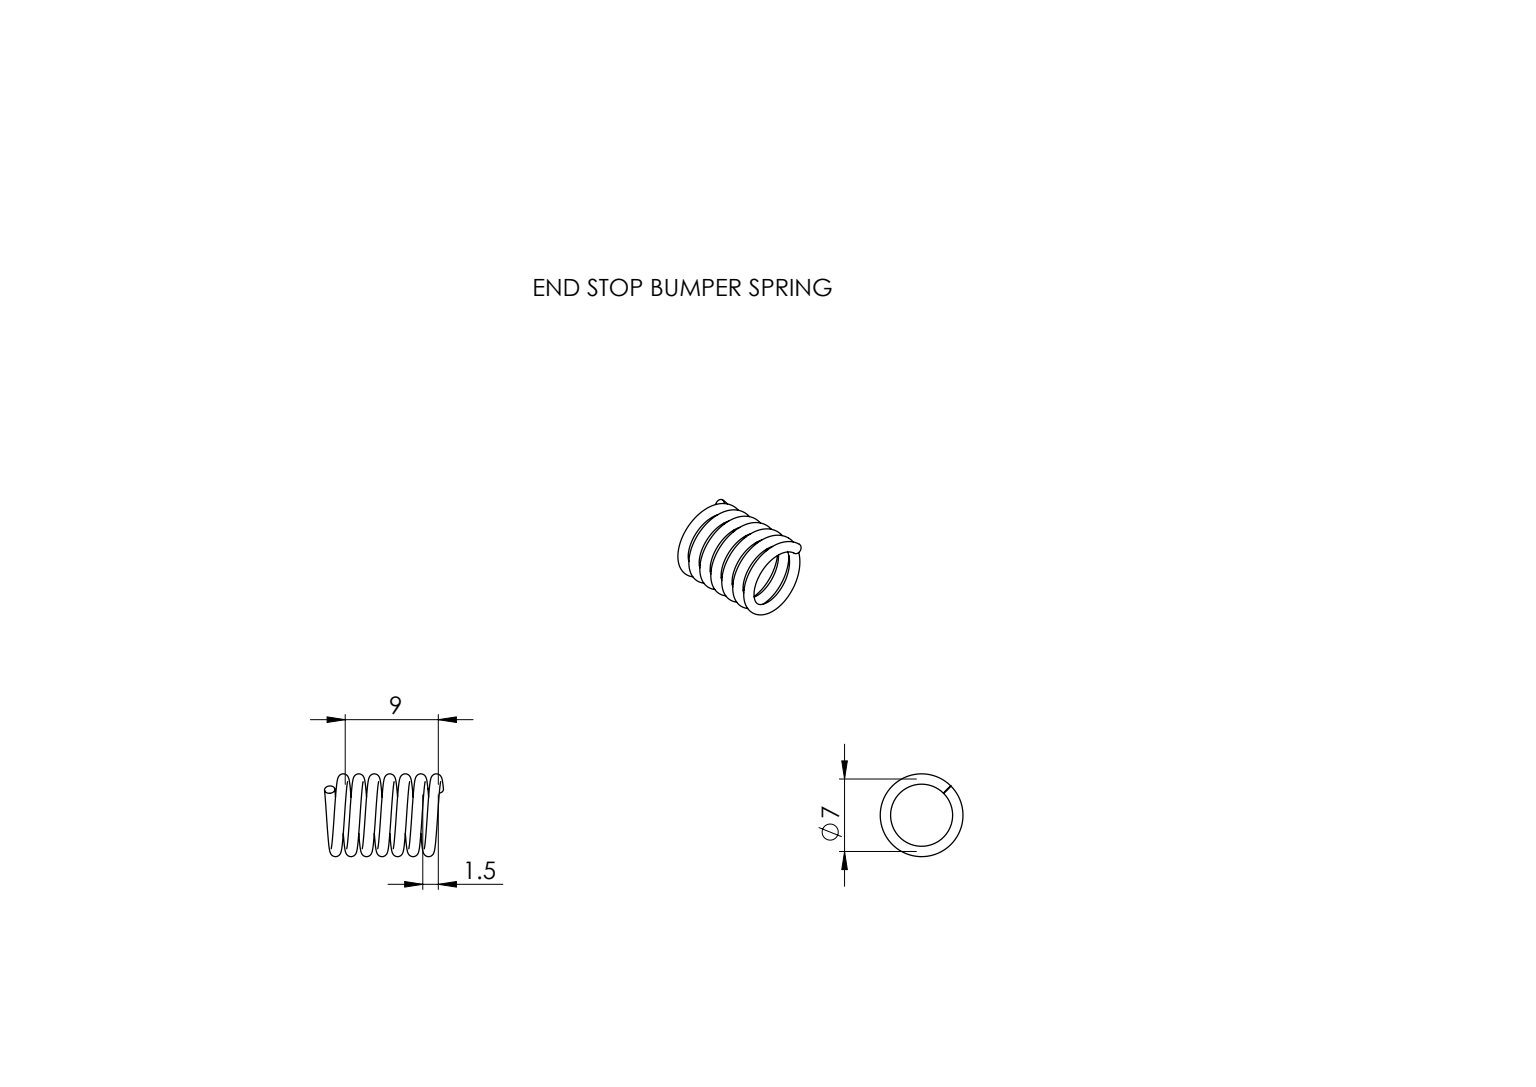
ISO-10303-21;
HEADER;
FILE_DESCRIPTION (('STEP AP214'),
    '1' );
FILE_NAME ('End Stop Bumper spring.step',
    '2026-10-08T13:46:47',
    ( '' ),
    ( '' ),
    'SwSTEP 2.0',
    'SolidWorks 2026',
    '' );
FILE_SCHEMA (( 'AUTOMOTIVE_DESIGN' ));
ENDSEC;

DATA;
#21=CARTESIAN_POINT ( 'NONE',  ( 57.71643183416158251, 13.97181229448536399, 16.72490539043799629 ) ) ;
#31=CARTESIAN_POINT ( 'NONE',  ( 51.40856816583843880, 12.97181229448534978, 13.68930817193506755 ) ) ;
#36=CARTESIAN_POINT ( 'NONE',  ( 52.87500000000000711, 7.878679656440349177, 12.87867965644035984 ) ) ;
#39=CARTESIAN_POINT ( 'NONE',  ( 51.09375000000000000, 11.24264068711927322, 11.99999999999998934 ) ) ;
#46=CARTESIAN_POINT ( 'NONE',  ( 51.56250000000000711, 6.999999999999997335, 15.00000000000000533 ) ) ;
#62=CARTESIAN_POINT ( 'NONE',  ( 52.25231816583844591, 7.219692298483957771, 17.87654654797633924 ) ) ;
#75=CARTESIAN_POINT ( 'NONE',  ( 53.43750000000000711, 10.00000000000001776, 18.99999999999999645 ) ) ;
#79=CARTESIAN_POINT ( 'NONE',  ( 56.84606816583843880, 8.411196891453267099, 19.02818770551464667 ) ) ;
#89=CARTESIAN_POINT ( 'NONE',  ( 52.27893183416158251, 8.411196891453236901, 10.97181229448535511 ) ) ;
#97=CARTESIAN_POINT ( 'NONE',  ( 53.25000000000000711, 7.878679656440361612, 17.12132034355964549 ) ) ;
#132=CARTESIAN_POINT ( 'NONE',  ( 56.49768183416158962, 12.87654654797631792, 12.21969229848393113 ) ) ;
#140=CARTESIAN_POINT ( 'NONE',  ( 50.84606816583843880, 8.825410453826357582, 18.02818770551464667 ) ) ;
#148=CARTESIAN_POINT ( 'NONE',  ( 52.59375000000000711, 11.24264068711927322, 11.99999999999998934 ) ) ;
#151=CARTESIAN_POINT ( 'NONE',  ( 53.53125000000000000, 11.24264068711929276, 18.00000000000000355 ) ) ;
#159=CARTESIAN_POINT ( 'NONE',  ( 56.53125000000000711, 11.24264068711929276, 18.00000000000000355 ) ) ;
#177=CARTESIAN_POINT ( 'NONE',  ( 52.43981816583844591, 10.06805114094564857, 19.00000000000000000 ) ) ;
#192=CARTESIAN_POINT ( 'NONE',  ( 58.59375000000000711, 11.65685424949236015, 10.99999999999998579 ) ) ;
#196=CARTESIAN_POINT ( 'NONE',  ( 54.97106816583843880, 5.971812294485345340, 13.41119689145326710 ) ) ;
#204=CARTESIAN_POINT ( 'NONE',  ( 56.49768183416158962, 12.87654654797631792, 12.21969229848393113 ) ) ;
#244=CARTESIAN_POINT ( 'NONE',  ( 55.93518183416157541, 9.931948859054379852, 18.99999999999999289 ) ) ;
#253=CARTESIAN_POINT ( 'NONE',  ( 54.56250000000000711, 6.999999999999997335, 15.00000000000000533 ) ) ;
#259=CARTESIAN_POINT ( 'NONE',  ( 59.96643183416158251, 7.028187705514638672, 13.68930817193508531 ) ) ;
#262=CARTESIAN_POINT ( 'NONE',  ( 54.28125000000000000, 8.757359312880703683, 11.99999999999999822 ) ) ;
#273=CARTESIAN_POINT ( 'NONE',  ( 56.15625000000002132, 7.000000000000003553, 16.24264068711929099 ) ) ;
#292=CARTESIAN_POINT ( 'NONE',  ( 59.00231816583843170, 12.07320092032949610, 12.83056023321021044 ) ) ;
#312=CARTESIAN_POINT ( 'NONE',  ( 54.37500000000000711, 7.171572875253794166, 12.17157287525381726 ) ) ;
#317=CARTESIAN_POINT ( 'NONE',  ( 51.78356816583844591, 8.275094609561968184, 11.02818770551464667 ) ) ;
#326=CARTESIAN_POINT ( 'NONE',  ( 53.21643183416158251, 13.97181229448536399, 16.72490539043799629 ) ) ;
#372=CARTESIAN_POINT ( 'NONE',  ( 57.18750000000000000, 9.999999999999978684, 10.99999999999999645 ) ) ;
#382=CARTESIAN_POINT ( 'NONE',  ( 53.43750000000000711, 10.00000000000000711, 17.99999999999999645 ) ) ;
#391=CARTESIAN_POINT ( 'NONE',  ( 55.65393183416158251, 6.971812294485357775, 16.17458954617365663 ) ) ;
#393=CARTESIAN_POINT ( 'NONE',  ( 55.21875000000000000, 13.00000000000000711, 16.24264068711927322 ) ) ;
#403=CARTESIAN_POINT ( 'NONE',  ( 56.31018183416157541, 12.99999999999999822, 15.06805114094562192 ) ) ;
#421=CARTESIAN_POINT ( 'NONE',  ( 54.97106816583843880, 5.971812294485345340, 13.41119689145326710 ) ) ;
#425=DIRECTION ( 'NONE',  ( 0.000000000000000000, 0.7071067811865414665, -0.7071067811865536790 ) ) ;
#440=CARTESIAN_POINT ( 'NONE',  ( 56.75231816583843170, 7.219692298483957771, 17.87654654797633924 ) ) ;
#450=CARTESIAN_POINT ( 'NONE',  ( 52.18518183416157541, 10.06805114094561659, 10.99999999999999645 ) ) ;
#454=DIRECTION ( 'NONE',  ( 0.06805114094563399774, -0.7054675904022866817, -0.7054675904022729149 ) ) ;
#493=CARTESIAN_POINT ( 'NONE',  ( 58.68750000000000000, 9.999999999999978684, 10.99999999999999645 ) ) ;
#501=CARTESIAN_POINT ( 'NONE',  ( 55.12500000000000711, 12.12132034355964727, 17.12132034355963484 ) ) ;
#508=CARTESIAN_POINT ( 'NONE',  ( 56.31018183416157541, 12.99999999999999822, 15.06805114094562192 ) ) ;
#517=CARTESIAN_POINT ( 'NONE',  ( 55.74768183416157541, 7.830560233210222876, 17.07320092032950498 ) ) ;
#534=CARTESIAN_POINT ( 'NONE',  ( 56.47106816583845301, 6.971812294485350670, 13.82541045382635403 ) ) ;
#560=CARTESIAN_POINT ( 'NONE',  ( 53.40393183416157541, 14.02818770551463956, 13.41119689145323335 ) ) ;
#568=CARTESIAN_POINT ( 'NONE',  ( 52.68750000000000711, 9.999999999999989342, 11.99999999999999467 ) ) ;
#605=CARTESIAN_POINT ( 'NONE',  ( 57.37500000000000000, 7.171572875253794166, 12.17157287525381726 ) ) ;
#608=ADVANCED_FACE ( 'NONE', ( #8331 ), #21063, .T. ) ;
#616=CARTESIAN_POINT ( 'NONE',  ( 58.50000000000000000, 12.12132034355963484, 12.87867965644034740 ) ) ;
#622=CARTESIAN_POINT ( 'NONE',  ( 54.15393183416158251, 6.971812294485357775, 16.17458954617365663 ) ) ;
#630=CARTESIAN_POINT ( 'NONE',  ( 59.87268183416157541, 7.926799079670491466, 12.83056023321021755 ) ) ;
#649=CARTESIAN_POINT ( 'NONE',  ( 53.93981816583844591, 10.06805114094563791, 17.99999999999999645 ) ) ;
#674=CARTESIAN_POINT ( 'NONE',  ( 57.09375000000000711, 11.65685424949236193, 10.99999999999998401 ) ) ;
#727=CARTESIAN_POINT ( 'NONE',  ( 58.21875000000000711, 14.00000000000000888, 16.65685424949235482 ) ) ;
#738=CARTESIAN_POINT ( 'NONE',  ( 55.50000000000000711, 12.12132034355963484, 12.87867965644034740 ) ) ;
#745=CARTESIAN_POINT ( 'NONE',  ( 57.62268183416157541, 12.07320092032950676, 17.16943976678977180 ) ) ;
#758=CARTESIAN_POINT ( 'NONE',  ( 59.77893183416158962, 8.825410453826341595, 11.97181229448535511 ) ) ;
#778=CARTESIAN_POINT ( 'NONE',  ( 54.12731816583844591, 12.16943976678978601, 17.07320092032949432 ) ) ;
#802=CARTESIAN_POINT ( 'NONE',  ( 58.68750000000000000, 9.999999999999978684, 10.99999999999999645 ) ) ;
#855=CARTESIAN_POINT ( 'NONE',  ( 55.27893183416158251, 8.825410453826341595, 11.97181229448535511 ) ) ;
#864=CARTESIAN_POINT ( 'NONE',  ( 58.46643183416158251, 7.028187705514638672, 13.68930817193508531 ) ) ;
#875=CARTESIAN_POINT ( 'NONE',  ( 57.03356816583845301, 11.31069182806492712, 17.97181229448534623 ) ) ;
#885=CARTESIAN_POINT ( 'NONE',  ( 56.00231816583843170, 12.07320092032949610, 12.83056023321021044 ) ) ;
#911=CARTESIAN_POINT ( 'NONE',  ( 54.37500000000000711, 7.171572875253794166, 12.17157287525381726 ) ) ;
#962=CARTESIAN_POINT ( 'NONE',  ( 51.75000000000000711, 7.878679656440361612, 17.12132034355964549 ) ) ;
#969=CARTESIAN_POINT ( 'NONE',  ( 60.62268183416157541, 12.78030770151606177, 17.87654654797631792 ) ) ;
#982=CARTESIAN_POINT ( 'NONE',  ( 58.65393183416157541, 5.971812294485358663, 16.58880310854675599 ) ) ;
#993=CARTESIAN_POINT ( 'NONE',  ( 50.28356816583843880, 8.275094609561968184, 11.02818770551464667 ) ) ;
#1003=CARTESIAN_POINT ( 'NONE',  ( 54.40856816583843880, 12.97181229448534978, 13.68930817193506755 ) ) ;
#1028=CARTESIAN_POINT ( 'NONE',  ( 58.78125000000000711, 8.343145750507600766, 11.00000000000000533 ) ) ;
#1086=CARTESIAN_POINT ( 'NONE',  ( 58.46643183416158251, 6.028187705514633343, 13.27509460956200016 ) ) ;
#1097=CARTESIAN_POINT ( 'NONE',  ( 60.71643183416158962, 13.97181229448536399, 16.72490539043799629 ) ) ;
#1107=CARTESIAN_POINT ( 'NONE',  ( 57.59606816583843880, 11.17458954617364242, 11.97181229448534800 ) ) ;
#1120=CARTESIAN_POINT ( 'NONE',  ( 50.93981816583844591, 10.06805114094563791, 17.99999999999999645 ) ) ;
#1148=CARTESIAN_POINT ( 'NONE',  ( 55.68750000000000000, 9.999999999999978684, 10.99999999999999645 ) ) ;
#1177=APPLICATION_CONTEXT ( 'automotive_design' ) ;
#1198=CARTESIAN_POINT ( 'NONE',  ( 51.37500000000000711, 7.878679656440349177, 12.87867965644035984 ) ) ;
#1205=CARTESIAN_POINT ( 'NONE',  ( 60.00000000000001421, 11.22198354879773419, 18.10280442057481665 ) ) ;
#1214=CARTESIAN_POINT ( 'NONE',  ( 59.68518183416157541, 10.06805114094561659, 10.99999999999999645 ) ) ;
#1223=CARTESIAN_POINT ( 'NONE',  ( 55.06481816583844591, 6.999999999999998224, 15.06805114094563436 ) ) ;
#1229=CARTESIAN_POINT ( 'NONE',  ( 59.34375000000000711, 8.757359312880723223, 18.00000000000000355 ) ) ;
#1231=CARTESIAN_POINT ( 'NONE',  ( 57.28125000000000711, 8.757359312880703683, 11.99999999999999822 ) ) ;
#1241=CARTESIAN_POINT ( 'NONE',  ( 59.25000000000000711, 7.878679656440361612, 17.12132034355964549 ) ) ;
#1257=CARTESIAN_POINT ( 'NONE',  ( 52.31250000000000711, 14.00000000000000000, 14.99999999999997691 ) ) ;
#1277=CARTESIAN_POINT ( 'NONE',  ( 51.56250000000000711, 5.999999999999996447, 15.00000000000001599 ) ) ;
#1295=CARTESIAN_POINT ( 'NONE',  ( 59.90625000000000711, 12.99999999999999645, 13.75735931288070191 ) ) ;
#1310=CARTESIAN_POINT ( 'NONE',  ( 51.18750000000000711, 9.999999999999989342, 11.99999999999999467 ) ) ;
#1328=CARTESIAN_POINT ( 'NONE',  ( 54.52893183416158962, 11.17458954617365663, 18.02818770551464311 ) ) ;
#1341=CARTESIAN_POINT ( 'NONE',  ( 50.65856816583843880, 6.028187705514649330, 16.72490539043803182 ) ) ;
#1348=CARTESIAN_POINT ( 'NONE',  ( 59.15625000000002132, 7.000000000000003553, 16.24264068711929099 ) ) ;
#1351=CARTESIAN_POINT ( 'NONE',  ( 51.50231816583844591, 12.07320092032949610, 12.83056023321021044 ) ) ;
#1360=CARTESIAN_POINT ( 'NONE',  ( 57.56250000000000000, 6.999999999999997335, 15.00000000000000533 ) ) ;
#1375=CARTESIAN_POINT ( 'NONE',  ( 56.93981816583843170, 10.06805114094564857, 19.00000000000000000 ) ) ;
#1387=CARTESIAN_POINT ( 'NONE',  ( 59.34375000000000711, 8.343145750507636293, 19.00000000000000000 ) ) ;
#1391=CARTESIAN_POINT ( 'NONE',  ( 57.68981816583843170, 9.931948859054346102, 10.99999999999999467 ) ) ;
#1410=CARTESIAN_POINT ( 'NONE',  ( 54.75000000000000711, 7.878679656440361612, 17.12132034355964549 ) ) ;
#1435=CARTESIAN_POINT ( 'NONE',  ( 60.00000000000002132, 13.28258829677531239, 17.07862169589594004 ) ) ;
#1449=CARTESIAN_POINT ( 'NONE',  ( 54.15393183416158251, 6.971812294485357775, 16.17458954617365663 ) ) ;
#1459=CARTESIAN_POINT ( 'NONE',  ( 51.12731816583844591, 12.16943976678978601, 17.07320092032949432 ) ) ;
#1469=CARTESIAN_POINT ( 'NONE',  ( 56.81250000000000000, 13.00000000000000000, 14.99999999999998757 ) ) ;
#1472=CARTESIAN_POINT ( 'NONE',  ( 50.18981816583844591, 9.931948859054354983, 11.99999999999999645 ) ) ;
#1478=VERTEX_POINT ( 'NONE', #10701 ) ;
#1482=CARTESIAN_POINT ( 'NONE',  ( 59.15625000000002132, 7.000000000000003553, 16.24264068711929099 ) ) ;
#1507=CARTESIAN_POINT ( 'NONE',  ( 51.84375000000001421, 8.343145750507638070, 19.00000000000000711 ) ) ;
#1523=CARTESIAN_POINT ( 'NONE',  ( 58.81481816583843170, 14.00000000000000178, 14.93194885905434610 ) ) ;
#1531=CARTESIAN_POINT ( 'NONE',  ( 52.93518183416157541, 9.931948859054372747, 17.99999999999999645 ) ) ;
#1540=CARTESIAN_POINT ( 'NONE',  ( 59.53125000000000711, 11.24264068711929276, 18.00000000000000000 ) ) ;
#1572=CARTESIAN_POINT ( 'NONE',  ( 56.21643183416158251, 13.97181229448536399, 16.72490539043799629 ) ) ;
#1583=CARTESIAN_POINT ( 'NONE',  ( 59.62500000000000711, 12.12132034355964727, 17.12132034355963484 ) ) ;
#1590=CARTESIAN_POINT ( 'NONE',  ( 54.65625000000001421, 7.000000000000003553, 16.24264068711929099 ) ) ;
#1592=CARTESIAN_POINT ( 'NONE',  ( 59.15625000000002132, 7.000000000000003553, 16.24264068711929099 ) ) ;
#1601=CARTESIAN_POINT ( 'NONE',  ( 55.50000000000000711, 12.12132034355963484, 12.87867965644034740 ) ) ;
#1621=CARTESIAN_POINT ( 'NONE',  ( 56.37731816583843170, 7.123453452023657206, 12.21969229848395599 ) ) ;
#1641=CARTESIAN_POINT ( 'NONE',  ( 53.62500000000000711, 12.82842712474620228, 17.82842712474617386 ) ) ;
#1650=CARTESIAN_POINT ( 'NONE',  ( 52.46643183416157541, 7.028187705514638672, 13.68930817193508531 ) ) ;
#1658=CARTESIAN_POINT ( 'NONE',  ( 56.71875000000000711, 13.00000000000000533, 16.24264068711927322 ) ) ;
#1688=CARTESIAN_POINT ( 'NONE',  ( 52.93518183416157541, 9.931948859054379852, 18.99999999999999289 ) ) ;
#1695=CARTESIAN_POINT ( 'NONE',  ( 58.87500000000000711, 7.878679656440349177, 12.87867965644035984 ) ) ;
#1703=CARTESIAN_POINT ( 'NONE',  ( 53.71875000000002132, 13.00000000000000711, 16.24264068711927322 ) ) ;
#1705=CARTESIAN_POINT ( 'NONE',  ( 52.78125000000000711, 8.757359312880703683, 11.99999999999999822 ) ) ;
#1713=CARTESIAN_POINT ( 'NONE',  ( 53.53125000000000000, 11.24264068711929276, 18.00000000000000355 ) ) ;
#1737=CARTESIAN_POINT ( 'NONE',  ( 55.34606816583843880, 8.411196891453267099, 19.02818770551464667 ) ) ;
#1740=SURFACE_STYLE_USAGE ( .BOTH. , #14468 ) ;
#1753=CARTESIAN_POINT ( 'NONE',  ( 55.87500000000000711, 7.171572875253794166, 12.17157287525381726 ) ) ;
#1757=CARTESIAN_POINT ( 'NONE',  ( 54.65625000000001421, 6.000000000000004441, 16.65685424949239390 ) ) ;
#1766=CARTESIAN_POINT ( 'NONE',  ( 57.81018183416157541, 14.00000000000000000, 15.06805114094561304 ) ) ;
#1774=CARTESIAN_POINT ( 'NONE',  ( 56.53125000000000711, 11.24264068711929276, 18.00000000000000000 ) ) ;
#1806=CARTESIAN_POINT ( 'NONE',  ( 53.21643183416158251, 13.97181229448536399, 16.72490539043799629 ) ) ;
#1814=CARTESIAN_POINT ( 'NONE',  ( 51.97106816583844591, 6.971812294485350670, 13.82541045382635403 ) ) ;
#1820=CARTESIAN_POINT ( 'NONE',  ( 55.12500000000000711, 12.12132034355964727, 17.12132034355963484 ) ) ;
#1824=CARTESIAN_POINT ( 'NONE',  ( 53.71875000000002132, 13.00000000000000711, 16.24264068711927322 ) ) ;
#1831=CARTESIAN_POINT ( 'NONE',  ( 51.93750000000000711, 10.00000000000000711, 17.99999999999999645 ) ) ;
#1851=CARTESIAN_POINT ( 'NONE',  ( 51.31481816583844591, 14.00000000000000178, 14.93194885905434610 ) ) ;
#1867=CARTESIAN_POINT ( 'NONE',  ( 53.90625000000000000, 13.99999999999999289, 13.34314575050759544 ) ) ;
#1872=CARTESIAN_POINT ( 'NONE',  ( 56.09606816583844591, 11.58880310854672935, 10.97181229448534445 ) ) ;
#1884=CARTESIAN_POINT ( 'NONE',  ( 55.27893183416158251, 8.411196891453236901, 10.97181229448535511 ) ) ;
#1893=CARTESIAN_POINT ( 'NONE',  ( 51.09375000000000711, 11.24264068711927322, 11.99999999999998934 ) ) ;
#1927=CARTESIAN_POINT ( 'NONE',  ( 58.27893183416158962, 8.411196891453236901, 10.97181229448535511 ) ) ;
#1936=CARTESIAN_POINT ( 'NONE',  ( 52.25231816583844591, 7.926799079670502124, 17.16943976678978245 ) ) ;
#1943=CARTESIAN_POINT ( 'NONE',  ( 54.28125000000000000, 8.757359312880703683, 11.99999999999999822 ) ) ;
#1946=CARTESIAN_POINT ( 'NONE',  ( 54.75000000000000711, 7.878679656440361612, 17.12132034355964549 ) ) ;
#1953=CARTESIAN_POINT ( 'NONE',  ( 52.31250000000000711, 13.00000000000000000, 14.99999999999998757 ) ) ;
#1968=CARTESIAN_POINT ( 'NONE',  ( 51.22106816583844591, 14.02818770551465377, 16.58880310854672757 ) ) ;
#1982=CARTESIAN_POINT ( 'NONE',  ( 59.06250000000000711, 5.999999999999996447, 15.00000000000001599 ) ) ;
#1986=CARTESIAN_POINT ( 'NONE',  ( 55.43981816583843170, 10.06805114094564857, 19.00000000000000000 ) ) ;
#1995=CARTESIAN_POINT ( 'NONE',  ( 59.15625000000002132, 6.000000000000004441, 16.65685424949239390 ) ) ;
#2002=CARTESIAN_POINT ( 'NONE',  ( 52.31250000000000711, 13.00000000000000000, 14.99999999999998757 ) ) ;
#2041=CARTESIAN_POINT ( 'NONE',  ( 54.15393183416158251, 5.971812294485358663, 16.58880310854675599 ) ) ;
#2047=CARTESIAN_POINT ( 'NONE',  ( 54.00000000000000711, 12.12132034355963484, 12.87867965644034740 ) ) ;
#2053=CARTESIAN_POINT ( 'NONE',  ( 55.68750000000000000, 9.999999999999989342, 11.99999999999999467 ) ) ;
#2066=CARTESIAN_POINT ( 'NONE',  ( 53.90625000000000000, 12.99999999999999645, 13.75735931288070191 ) ) ;
#2084=CARTESIAN_POINT ( 'NONE',  ( 53.75231816583844591, 7.219692298483957771, 17.87654654797633924 ) ) ;
#2088=EDGE_CURVE ( 'NONE', #16693, #10540, #5521, .T. ) ;
#2099=CARTESIAN_POINT ( 'NONE',  ( 57.28125000000000711, 8.343145750507600766, 11.00000000000000355 ) ) ;
#2103=CARTESIAN_POINT ( 'NONE',  ( 53.00231816583844591, 12.78030770151603868, 12.12345345202365188 ) ) ;
#2114=CARTESIAN_POINT ( 'NONE',  ( 54.99768183416157541, 12.87654654797631792, 12.21969229848393113 ) ) ;
#2126=EDGE_LOOP ( 'NONE', ( #8202, #17901 ) ) ;
#2156=CARTESIAN_POINT ( 'NONE',  ( 57.84375000000000711, 8.343145750507638070, 19.00000000000000711 ) ) ;
#2166=CARTESIAN_POINT ( 'NONE',  ( 55.87500000000000711, 7.878679656440349177, 12.87867965644035984 ) ) ;
#2176=CARTESIAN_POINT ( 'NONE',  ( 59.02893183416158251, 11.17458954617365663, 18.02818770551464311 ) ) ;
#2179=CARTESIAN_POINT ( 'NONE',  ( 54.93750000000000711, 10.00000000000000711, 17.99999999999999645 ) ) ;
#2189=CARTESIAN_POINT ( 'NONE',  ( 58.37268183416157541, 7.926799079670491466, 12.83056023321021755 ) ) ;
#2208=CARTESIAN_POINT ( 'NONE',  ( 53.37731816583844591, 7.123453452023657206, 12.21969229848395599 ) ) ;
#2224=CARTESIAN_POINT ( 'NONE',  ( 52.68750000000000711, 9.999999999999978684, 10.99999999999999645 ) ) ;
#2228=CARTESIAN_POINT ( 'NONE',  ( 52.90856816583843880, 13.97181229448534978, 13.27509460956196641 ) ) ;
#2240=CARTESIAN_POINT ( 'NONE',  ( 59.81250000000000711, 14.00000000000000000, 14.99999999999997691 ) ) ;
#2279=STYLED_ITEM ( 'NONE', ( #5346 ), #22323 ) ;
#2287=CARTESIAN_POINT ( 'NONE',  ( 59.15625000000002132, 6.000000000000004441, 16.65685424949239390 ) ) ;
#2297=CARTESIAN_POINT ( 'NONE',  ( 56.15625000000002132, 7.000000000000003553, 16.24264068711929099 ) ) ;
#2304=CARTESIAN_POINT ( 'NONE',  ( 58.46643183416158251, 7.028187705514638672, 13.68930817193508531 ) ) ;
#2317=CARTESIAN_POINT ( 'NONE',  ( 58.93518183416157541, 9.931948859054372747, 17.99999999999999645 ) ) ;
#2333=CARTESIAN_POINT ( 'NONE',  ( 58.06481816583843170, 6.999999999999998224, 15.06805114094563436 ) ) ;
#2360=CARTESIAN_POINT ( 'NONE',  ( 55.37268183416157541, 7.219692298483935566, 12.12345345202367675 ) ) ;
#2403=CARTESIAN_POINT ( 'NONE',  ( 55.96875000000000000, 5.999999999999987566, 13.34314575050763452 ) ) ;
#2411=CARTESIAN_POINT ( 'NONE',  ( 57.93750000000000000, 10.00000000000000711, 17.99999999999999645 ) ) ;
#2418=CARTESIAN_POINT ( 'NONE',  ( 59.77893183416158962, 8.825410453826341595, 11.97181229448535511 ) ) ;
#2427=CARTESIAN_POINT ( 'NONE',  ( 60.99768183416157541, 12.16943976678977535, 12.92679907967048614 ) ) ;
#2445=CARTESIAN_POINT ( 'NONE',  ( 57.12731816583843170, 12.16943976678978601, 17.07320092032949432 ) ) ;
#2472=CARTESIAN_POINT ( 'NONE',  ( 53.15625000000001421, 6.000000000000004441, 16.65685424949239390 ) ) ;
#2518=CARTESIAN_POINT ( 'NONE',  ( 59.90625000000000711, 13.99999999999999289, 13.34314575050759544 ) ) ;
#2522=EDGE_LOOP ( 'NONE', ( #4591, #11690 ) ) ;
#2525=CARTESIAN_POINT ( 'NONE',  ( 57.09375000000000711, 11.24264068711927322, 11.99999999999998934 ) ) ;
#2531=CARTESIAN_POINT ( 'NONE',  ( 58.56018183416157541, 7.000000000000000000, 14.93194885905437097 ) ) ;
#2540=CARTESIAN_POINT ( 'NONE',  ( 56.49768183416158962, 12.16943976678977535, 12.92679907967048614 ) ) ;
#2557=CARTESIAN_POINT ( 'NONE',  ( 56.84606816583843880, 8.825410453826357582, 18.02818770551464667 ) ) ;
#2575=CARTESIAN_POINT ( 'NONE',  ( 52.03125000000000711, 11.65685424949239923, 18.99999999999998934 ) ) ;
#2587=CARTESIAN_POINT ( 'NONE',  ( 56.25000000000000711, 7.171572875253819923, 17.82842712474619873 ) ) ;
#2657=CARTESIAN_POINT ( 'NONE',  ( 57.90393183416158251, 13.02818770551463778, 13.82541045382633982 ) ) ;
#2668=CARTESIAN_POINT ( 'NONE',  ( 59.31018183416157541, 12.99999999999999822, 15.06805114094562192 ) ) ;
#2682=CARTESIAN_POINT ( 'NONE',  ( 57.31481816583843170, 12.99999999999999822, 14.93194885905435676 ) ) ;
#2691=CARTESIAN_POINT ( 'NONE',  ( 57.68981816583843170, 9.931948859054354983, 11.99999999999999645 ) ) ;
#2713=CARTESIAN_POINT ( 'NONE',  ( 54.46875000000000000, 5.999999999999987566, 13.34314575050763452 ) ) ;
#2770=CARTESIAN_POINT ( 'NONE',  ( 53.02893183416157541, 11.17458954617365663, 18.02818770551464311 ) ) ;
#2771=CARTESIAN_POINT ( 'NONE',  ( 60.00000000000002132, 12.52638886096845816, 13.34932382114196692 ) ) ;
#2780=CARTESIAN_POINT ( 'NONE',  ( 59.40393183416158251, 14.02818770551463956, 13.41119689145323335 ) ) ;
#2791=CARTESIAN_POINT ( 'NONE',  ( 56.18981816583843170, 9.931948859054354983, 11.99999999999999645 ) ) ;
#2803=CARTESIAN_POINT ( 'NONE',  ( 54.97106816583843880, 6.971812294485350670, 13.82541045382635403 ) ) ;
#2827=CARTESIAN_POINT ( 'NONE',  ( 53.53125000000000000, 11.65685424949239923, 18.99999999999998934 ) ) ;
#2881=CARTESIAN_POINT ( 'NONE',  ( 58.37268183416157541, 7.219692298483935566, 12.12345345202367675 ) ) ;
#2893=CARTESIAN_POINT ( 'NONE',  ( 54.71643183416158251, 12.97181229448535689, 16.31069182806490758 ) ) ;
#2904=CARTESIAN_POINT ( 'NONE',  ( 58.15856816583844591, 7.028187705514647554, 16.31069182806492179 ) ) ;
#2910=CARTESIAN_POINT ( 'NONE',  ( 56.34375000000000711, 8.757359312880723223, 18.00000000000000355 ) ) ;
#2913=CARTESIAN_POINT ( 'NONE',  ( 51.68981816583844591, 9.931948859054354983, 11.99999999999999645 ) ) ;
#2940=CARTESIAN_POINT ( 'NONE',  ( 53.81250000000000711, 14.00000000000000000, 14.99999999999997691 ) ) ;
#3003=CARTESIAN_POINT ( 'NONE',  ( 60.00000000000005684, 13.02863400130356375, 14.80978507604997851 ) ) ;
#3013=CARTESIAN_POINT ( 'NONE',  ( 54.81018183416157541, 12.99999999999999822, 15.06805114094562192 ) ) ;
#3023=ORIENTED_EDGE ( 'NONE', *, *, #17689, .T. ) ;
#3024=CARTESIAN_POINT ( 'NONE',  ( 59.00231816583843170, 12.07320092032949610, 12.83056023321021044 ) ) ;
#3026=MECHANICAL_DESIGN_GEOMETRIC_PRESENTATION_REPRESENTATION('',(#8030),#3797);
#3040=CARTESIAN_POINT ( 'NONE',  ( 59.34375000000000711, 8.757359312880723223, 18.00000000000000355 ) ) ;
#3072=CARTESIAN_POINT ( 'NONE',  ( 56.47106816583845301, 5.971812294485345340, 13.41119689145326710 ) ) ;
#3087=CARTESIAN_POINT ( 'NONE',  ( 59.81250000000000711, 14.00000000000000000, 14.99999999999997691 ) ) ;
#3091=CARTESIAN_POINT ( 'NONE',  ( 54.93750000000000711, 10.00000000000001776, 18.99999999999999645 ) ) ;
#3109=CARTESIAN_POINT ( 'NONE',  ( 59.15625000000001421, 7.000000000000002665, 16.24264068711929099 ) ) ;
#3111=CARTESIAN_POINT ( 'NONE',  ( 0.000000000000000000, 0.000000000000000000, 0.000000000000000000 ) ) ;
#3137=CARTESIAN_POINT ( 'NONE',  ( 60.90393183416158962, 14.02818770551463956, 13.41119689145323335 ) ) ;
#3146=CARTESIAN_POINT ( 'NONE',  ( 54.78356816583844591, 8.689308171935074654, 12.02818770551464489 ) ) ;
#3152=CARTESIAN_POINT ( 'NONE',  ( 58.03125000000000711, 11.24264068711929276, 18.00000000000000355 ) ) ;
#3154=CARTESIAN_POINT ( 'NONE',  ( 60.00000000000000711, 12.12132034355963484, 12.87867965644034740 ) ) ;
#3162=CARTESIAN_POINT ( 'NONE',  ( 57.65625000000002132, 7.000000000000003553, 16.24264068711929099 ) ) ;
#3163=SURFACE_SIDE_STYLE ('',( #8345 ) ) ;
#3183=CARTESIAN_POINT ( 'NONE',  ( 56.84606816583843880, 8.411196891453267099, 19.02818770551464667 ) ) ;
#3198=CARTESIAN_POINT ( 'NONE',  ( 59.53125000000000711, 11.65685424949239923, 18.99999999999998934 ) ) ;
#3202=CARTESIAN_POINT ( 'NONE',  ( 55.40625000000000000, 13.99999999999999289, 13.34314575050759544 ) ) ;
#3219=CARTESIAN_POINT ( 'NONE',  ( 56.06250000000000000, 6.999999999999997335, 15.00000000000000533 ) ) ;
#3231=ORIENTED_EDGE ( 'NONE', *, *, #2088, .F. ) ;
#3246=CARTESIAN_POINT ( 'NONE',  ( 59.99999999999182165, 10.93426768979392349, 18.41713329524482390 ) ) ;
#3255=CARTESIAN_POINT ( 'NONE',  ( 59.59143183416158962, 11.72490539043799984, 11.02818770551463246 ) ) ;
#3267=CARTESIAN_POINT ( 'NONE',  ( 53.37731816583844591, 7.830560233210212218, 12.92679907967049679 ) ) ;
#3276=CARTESIAN_POINT ( 'NONE',  ( 55.96875000000000000, 6.999999999999992895, 13.75735931288071967 ) ) ;
#3278=CARTESIAN_POINT ( 'NONE',  ( 57.93750000000000000, 10.00000000000000711, 17.99999999999999645 ) ) ;
#3287=CARTESIAN_POINT ( 'NONE',  ( 58.68750000000000000, 9.999999999999989342, 11.99999999999999467 ) ) ;
#3294=FACE_OUTER_BOUND ( 'NONE', #10599, .T. ) ;
#3304=CARTESIAN_POINT ( 'NONE',  ( 51.37500000000000711, 7.171572875253794166, 12.17157287525381726 ) ) ;
#3321=CARTESIAN_POINT ( 'NONE',  ( 51.93750000000000711, 10.00000000000001776, 18.99999999999999645 ) ) ;
#3332=CARTESIAN_POINT ( 'NONE',  ( 60.24768183416157541, 7.123453452023678523, 17.78030770151605822 ) ) ;
#3342=CARTESIAN_POINT ( 'NONE',  ( 57.00000000000000000, 12.12132034355963484, 12.87867965644034740 ) ) ;
#3364=CARTESIAN_POINT ( 'NONE',  ( 60.00000000000000711, 12.67839003132778686, 16.61512380723988258 ) ) ;
#3378=CARTESIAN_POINT ( 'NONE',  ( 56.96643183416158251, 6.028187705514633343, 13.27509460956200016 ) ) ;
#3386=CARTESIAN_POINT ( 'NONE',  ( 59.90625000000000711, 12.99999999999999645, 13.75735931288070191 ) ) ;
#3393=CARTESIAN_POINT ( 'NONE',  ( 55.78125000000000000, 8.757359312880703683, 11.99999999999999822 ) ) ;
#3395=CARTESIAN_POINT ( 'NONE',  ( 50.37731816583844591, 7.830560233210212218, 12.92679907967049679 ) ) ;
#3429=CARTESIAN_POINT ( 'NONE',  ( 59.00231816583843170, 12.78030770151603868, 12.12345345202365188 ) ) ;
#3449=CARTESIAN_POINT ( 'NONE',  ( 53.53125000000000000, 11.65685424949239923, 18.99999999999998934 ) ) ;
#3458=CARTESIAN_POINT ( 'NONE',  ( 57.15393183416157541, 5.971812294485358663, 16.58880310854675599 ) ) ;
#3466=CARTESIAN_POINT ( 'NONE',  ( 54.65625000000000711, 7.000000000000002665, 16.24264068711929099 ) ) ;
#3488=CARTESIAN_POINT ( 'NONE',  ( 60.00000000000001421, 11.91318284588047405, 17.59430459896656629 ) ) ;
#3499=CARTESIAN_POINT ( 'NONE',  ( 53.31018183416157541, 14.00000000000000000, 15.06805114094561304 ) ) ;
#3508=CARTESIAN_POINT ( 'NONE',  ( 54.12731816583844591, 12.16943976678978601, 17.07320092032949432 ) ) ;
#3515=CARTESIAN_POINT ( 'NONE',  ( 55.50000000000000711, 12.12132034355963484, 12.87867965644034740 ) ) ;
#3517=CARTESIAN_POINT ( 'NONE',  ( 56.15625000000002132, 7.000000000000003553, 16.24264068711929099 ) ) ;
#3525=CARTESIAN_POINT ( 'NONE',  ( 52.59375000000000711, 11.24264068711927322, 11.99999999999998934 ) ) ;
#3542=CARTESIAN_POINT ( 'NONE',  ( 55.81481816583843170, 14.00000000000000178, 14.93194885905434610 ) ) ;
#3554=CARTESIAN_POINT ( 'NONE',  ( 58.87500000000000711, 7.171572875253794166, 12.17157287525381726 ) ) ;
#3559=CARTESIAN_POINT ( 'NONE',  ( 51.37500000000000711, 7.171572875253794166, 12.17157287525381726 ) ) ;
#3569=CARTESIAN_POINT ( 'NONE',  ( 59.40393183416158251, 14.02818770551463956, 13.41119689145323335 ) ) ;
#3577=CARTESIAN_POINT ( 'NONE',  ( 58.68750000000000000, 9.999999999999989342, 11.99999999999999467 ) ) ;
#3605=CARTESIAN_POINT ( 'NONE',  ( 52.46643183416157541, 6.028187705514633343, 13.27509460956200016 ) ) ;
#3613=CARTESIAN_POINT ( 'NONE',  ( 53.09606816583843170, 11.17458954617364242, 11.97181229448534800 ) ) ;
#3620=CARTESIAN_POINT ( 'NONE',  ( 53.15625000000001421, 7.000000000000003553, 16.24264068711929099 ) ) ;
#3623=CARTESIAN_POINT ( 'NONE',  ( 52.12500000000000711, 12.12132034355964727, 17.12132034355963484 ) ) ;
#3631=CARTESIAN_POINT ( 'NONE',  ( 54.46875000000000000, 6.999999999999992895, 13.75735931288071967 ) ) ;
#3651=CARTESIAN_POINT ( 'NONE',  ( 51.78356816583844591, 8.275094609561968184, 11.02818770551464667 ) ) ;
#3667=CARTESIAN_POINT ( 'NONE',  ( 54.00000000000000711, 12.82842712474617741, 12.17157287525379239 ) ) ;
#3671=CARTESIAN_POINT ( 'NONE',  ( 51.97106816583844591, 5.971812294485345340, 13.41119689145326710 ) ) ;
#3679=CARTESIAN_POINT ( 'NONE',  ( 52.37268183416157541, 7.219692298483935566, 12.12345345202367675 ) ) ;
#3686=CARTESIAN_POINT ( 'NONE',  ( 51.46875000000000711, 6.999999999999992006, 13.75735931288071967 ) ) ;
#3719=CARTESIAN_POINT ( 'NONE',  ( 57.43518183416157541, 9.931948859054379852, 18.99999999999999289 ) ) ;
#3729=CARTESIAN_POINT ( 'NONE',  ( 54.22106816583844591, 13.02818770551464489, 16.17458954617363531 ) ) ;
#3736=CARTESIAN_POINT ( 'NONE',  ( 51.18750000000000711, 9.999999999999989342, 11.99999999999999467 ) ) ;
#3740=CARTESIAN_POINT ( 'NONE',  ( 53.62500000000000711, 12.12132034355964727, 17.12132034355963484 ) ) ;
#3747=CARTESIAN_POINT ( 'NONE',  ( 53.34375000000000000, 8.757359312880723223, 18.00000000000000355 ) ) ;
#3770=CARTESIAN_POINT ( 'NONE',  ( 52.06481816583844591, 5.999999999999996447, 15.06805114094564502 ) ) ;
#3787=CARTESIAN_POINT ( 'NONE',  ( 58.12500000000000000, 12.82842712474620228, 17.82842712474617386 ) ) ;
#3792=CARTESIAN_POINT ( 'NONE',  ( 55.15856816583844591, 6.028187705514649330, 16.72490539043803182 ) ) ;
#3797=( GEOMETRIC_REPRESENTATION_CONTEXT ( 3 ) GLOBAL_UNCERTAINTY_ASSIGNED_CONTEXT ( ( #17687 ) ) GLOBAL_UNIT_ASSIGNED_CONTEXT ( ( #19455, #6773, #14089 ) ) REPRESENTATION_CONTEXT ( 'NONE', 'WORKASPACE' ) );
#3804=APPLICATION_CONTEXT ( 'automotive_design' ) ;
#3806=CARTESIAN_POINT ( 'NONE',  ( 60.00000000000000711, 12.82842712474617741, 12.17157287525379239 ) ) ;
#3815=CARTESIAN_POINT ( 'NONE',  ( 51.37500000000000711, 7.878679656440349177, 12.87867965644035984 ) ) ;
#3851=CARTESIAN_POINT ( 'NONE',  ( 55.27893183416158251, 8.411196891453236901, 10.97181229448535511 ) ) ;
#3859=CARTESIAN_POINT ( 'NONE',  ( 57.56250000000000000, 6.999999999999997335, 15.00000000000000533 ) ) ;
#3865=CARTESIAN_POINT ( 'NONE',  ( 54.93750000000000711, 10.00000000000000711, 17.99999999999999645 ) ) ;
#3868=CARTESIAN_POINT ( 'NONE',  ( 51.28125000000000000, 8.757359312880703683, 11.99999999999999822 ) ) ;
#3875=CARTESIAN_POINT ( 'NONE',  ( 52.96875000000000000, 6.999999999999992895, 13.75735931288071967 ) ) ;
#3889=CARTESIAN_POINT ( 'NONE',  ( 50.28356816583843880, 8.275094609561968184, 11.02818770551464667 ) ) ;
#3904=CARTESIAN_POINT ( 'NONE',  ( 55.50000000000000711, 12.82842712474617741, 12.17157287525379239 ) ) ;
#3907=CARTESIAN_POINT ( 'NONE',  ( 52.34606816583843880, 8.411196891453267099, 19.02818770551464667 ) ) ;
#3915=CARTESIAN_POINT ( 'NONE',  ( 56.77893183416158251, 8.411196891453236901, 10.97181229448535511 ) ) ;
#3965=CARTESIAN_POINT ( 'NONE',  ( 59.25000000000000711, 7.171572875253819923, 17.82842712474619873 ) ) ;
#3967=SHAPE_DEFINITION_REPRESENTATION ( #22514, #10226 ) ;
#3975=CARTESIAN_POINT ( 'NONE',  ( 58.40625000000000711, 12.99999999999999645, 13.75735931288070191 ) ) ;
#3981=CARTESIAN_POINT ( 'NONE',  ( 54.46875000000000000, 6.999999999999992895, 13.75735931288071967 ) ) ;
#3992=CARTESIAN_POINT ( 'NONE',  ( 58.09143183416158962, 11.31069182806491291, 12.02818770551463778 ) ) ;
#4011=CARTESIAN_POINT ( 'NONE',  ( 58.43981816583843170, 10.06805114094563791, 17.99999999999999645 ) ) ;
#4027=CARTESIAN_POINT ( 'NONE',  ( 58.31250000000000000, 14.00000000000000000, 14.99999999999997691 ) ) ;
#4031=CARTESIAN_POINT ( 'NONE',  ( 54.03356816583844591, 11.72490539043803004, 18.97181229448534268 ) ) ;
#4043=CARTESIAN_POINT ( 'NONE',  ( 52.56018183416157541, 5.999999999999996447, 14.93194885905437808 ) ) ;
#4051=CARTESIAN_POINT ( 'NONE',  ( 51.75000000000000711, 7.878679656440361612, 17.12132034355964549 ) ) ;
#4084=CARTESIAN_POINT ( 'NONE',  ( 58.87500000000000711, 7.171572875253794166, 12.17157287525381726 ) ) ;
#4092=CARTESIAN_POINT ( 'NONE',  ( 52.96875000000000000, 6.999999999999992895, 13.75735931288071967 ) ) ;
#4101=CARTESIAN_POINT ( 'NONE',  ( 55.37268183416157541, 7.926799079670491466, 12.83056023321021755 ) ) ;
#4113=CARTESIAN_POINT ( 'NONE',  ( 55.93518183416157541, 9.931948859054372747, 17.99999999999999645 ) ) ;
#4132=CARTESIAN_POINT ( 'NONE',  ( 55.06481816583844591, 5.999999999999996447, 15.06805114094564502 ) ) ;
#4151=CARTESIAN_POINT ( 'NONE',  ( 52.15856816583843880, 6.028187705514649330, 16.72490539043803182 ) ) ;
#4160=CIRCLE ( 'NONE', #16028, 0.5000000000000006661 ) ;
#4161=CARTESIAN_POINT ( 'NONE',  ( 56.12268183416157541, 12.78030770151606177, 17.87654654797631792 ) ) ;
#4208=CARTESIAN_POINT ( 'NONE',  ( 57.93750000000000000, 10.00000000000001776, 18.99999999999999645 ) ) ;
#4219=CARTESIAN_POINT ( 'NONE',  ( 53.25000000000000711, 7.878679656440361612, 17.12132034355964549 ) ) ;
#4226=CARTESIAN_POINT ( 'NONE',  ( 54.71643183416158251, 12.97181229448535689, 16.31069182806490758 ) ) ;
#4237=CARTESIAN_POINT ( 'NONE',  ( 57.43518183416157541, 9.931948859054372747, 17.99999999999999645 ) ) ;
#4241=ADVANCED_FACE ( 'NONE', ( #4639 ), #20680, .F. ) ;
#4257=CARTESIAN_POINT ( 'NONE',  ( 57.31481816583843170, 12.99999999999999822, 14.93194885905435676 ) ) ;
#4271=CARTESIAN_POINT ( 'NONE',  ( 52.12500000000000711, 12.82842712474620228, 17.82842712474617386 ) ) ;
#4282=CARTESIAN_POINT ( 'NONE',  ( 55.96875000000000000, 5.999999999999987566, 13.34314575050763452 ) ) ;
#4323=CARTESIAN_POINT ( 'NONE',  ( 55.50000000000000711, 12.82842712474617741, 12.17157287525379239 ) ) ;
#4331=CARTESIAN_POINT ( 'NONE',  ( 55.78125000000000000, 8.757359312880703683, 11.99999999999999822 ) ) ;
#4338=CARTESIAN_POINT ( 'NONE',  ( 59.68518183416157541, 10.06805114094562548, 11.99999999999999645 ) ) ;
#4339=CARTESIAN_POINT ( 'NONE',  ( 60.00000000000000000, 12.92210812677098275, 14.19519413938285268 ) ) ;
#4349=CARTESIAN_POINT ( 'NONE',  ( 60.43518183416157541, 9.931948859054372747, 17.99999999999999645 ) ) ;
#4368=CARTESIAN_POINT ( 'NONE',  ( 56.56481816583843170, 6.999999999999998224, 15.06805114094563436 ) ) ;
#4396=CARTESIAN_POINT ( 'NONE',  ( 57.56250000000000000, 5.999999999999996447, 15.00000000000001599 ) ) ;
#4450=CARTESIAN_POINT ( 'NONE',  ( 51.65625000000000711, 7.000000000000003553, 16.24264068711929099 ) ) ;
#4455=CARTESIAN_POINT ( 'NONE',  ( 57.52893183416158962, 11.17458954617365663, 18.02818770551464311 ) ) ;
#4464=CARTESIAN_POINT ( 'NONE',  ( 58.74768183416157541, 7.830560233210222876, 17.07320092032950498 ) ) ;
#4484=CARTESIAN_POINT ( 'NONE',  ( 55.53356816583845301, 11.31069182806492712, 17.97181229448534623 ) ) ;
#4514=CARTESIAN_POINT ( 'NONE',  ( 55.03125000000000000, 11.65685424949239923, 18.99999999999998934 ) ) ;
#4574=CARTESIAN_POINT ( 'NONE',  ( 51.09375000000000000, 11.24264068711927322, 11.99999999999998934 ) ) ;
#4581=CARTESIAN_POINT ( 'NONE',  ( 56.96643183416158251, 7.028187705514638672, 13.68930817193508531 ) ) ;
#4591=ORIENTED_EDGE ( 'NONE', *, *, #8075, .F. ) ;
#4592=CARTESIAN_POINT ( 'NONE',  ( 52.65393183416158251, 6.971812294485357775, 16.17458954617365663 ) ) ;
#4604=CARTESIAN_POINT ( 'NONE',  ( 58.72106816583844591, 13.02818770551464489, 16.17458954617363531 ) ) ;
#4615=CARTESIAN_POINT ( 'NONE',  ( 52.43981816583844591, 10.06805114094563791, 17.99999999999999645 ) ) ;
#4628=CARTESIAN_POINT ( 'NONE',  ( 51.75000000000000711, 7.171572875253819923, 17.82842712474619873 ) ) ;
#4637=CARTESIAN_POINT ( 'NONE',  ( 58.87500000000000711, 7.171572875253794166, 12.17157287525381726 ) ) ;
#4639=FACE_OUTER_BOUND ( 'NONE', #2126, .T. ) ;
#4694=CARTESIAN_POINT ( 'NONE',  ( 60.15393183416158962, 5.971812294485358663, 16.58880310854675599 ) ) ;
#4706=CARTESIAN_POINT ( 'NONE',  ( 52.37268183416157541, 7.926799079670491466, 12.83056023321021755 ) ) ;
#4716=CARTESIAN_POINT ( 'NONE',  ( 57.87731816583843170, 7.830560233210212218, 12.92679907967049679 ) ) ;
#4722=CARTESIAN_POINT ( 'NONE',  ( 58.59375000000000711, 11.24264068711927322, 11.99999999999998934 ) ) ;
#4726=CARTESIAN_POINT ( 'NONE',  ( 57.87731816583843170, 7.830560233210212218, 12.92679907967049679 ) ) ;
#4750=CARTESIAN_POINT ( 'NONE',  ( 53.34375000000000000, 8.343145750507638070, 19.00000000000000711 ) ) ;
#4807=CARTESIAN_POINT ( 'NONE',  ( 59.99999999999995026, 12.78483204250637328, 17.66020603153145885 ) ) ;
#4818=CARTESIAN_POINT ( 'NONE',  ( 53.40393183416157541, 13.02818770551463778, 13.82541045382633982 ) ) ;
#4828=CARTESIAN_POINT ( 'NONE',  ( 57.22106816583844591, 13.02818770551464489, 16.17458954617363531 ) ) ;
#4836=CARTESIAN_POINT ( 'NONE',  ( 59.81250000000000711, 13.00000000000000000, 14.99999999999998757 ) ) ;
#4839=CARTESIAN_POINT ( 'NONE',  ( 51.40856816583843880, 12.97181229448534978, 13.68930817193506755 ) ) ;
#4868=CARTESIAN_POINT ( 'NONE',  ( 58.43981816583843170, 10.06805114094564857, 19.00000000000000000 ) ) ;
#4887=CARTESIAN_POINT ( 'NONE',  ( 51.09375000000000000, 11.65685424949236193, 10.99999999999998401 ) ) ;
#4929=CARTESIAN_POINT ( 'NONE',  ( 60.00000000000000000, 13.23725887712638283, 12.63247214140022123 ) ) ;
#4940=CARTESIAN_POINT ( 'NONE',  ( 60.24768183416157541, 7.123453452023678523, 17.78030770151605822 ) ) ;
#4952=CARTESIAN_POINT ( 'NONE',  ( 51.50231816583844591, 12.78030770151603868, 12.12345345202365188 ) ) ;
#4966=CARTESIAN_POINT ( 'NONE',  ( 50.75231816583844591, 7.926799079670502124, 17.16943976678978245 ) ) ;
#4995=CARTESIAN_POINT ( 'NONE',  ( 58.72106816583844591, 14.02818770551465377, 16.58880310854672757 ) ) ;
#4996=EDGE_CURVE ( 'NONE', #16693, #8676, #18626, .T. ) ;
#5010=CARTESIAN_POINT ( 'NONE',  ( 59.62500000000000711, 12.82842712474620228, 17.82842712474617386 ) ) ;
#5014=CARTESIAN_POINT ( 'NONE',  ( 57.97106816583845301, 5.971812294485345340, 13.41119689145326710 ) ) ;
#5029=CARTESIAN_POINT ( 'NONE',  ( 56.81250000000000000, 13.00000000000000000, 14.99999999999998757 ) ) ;
#5047=CARTESIAN_POINT ( 'NONE',  ( 60.00000000000002132, 13.01044786497014805, 14.65336842865874267 ) ) ;
#5056=CARTESIAN_POINT ( 'NONE',  ( 53.49768183416157541, 12.16943976678977535, 12.92679907967048614 ) ) ;
#5066=CARTESIAN_POINT ( 'NONE',  ( 57.50231816583843170, 12.07320092032949610, 12.83056023321021044 ) ) ;
#5074=CARTESIAN_POINT ( 'NONE',  ( 56.25000000000000711, 7.878679656440361612, 17.12132034355964549 ) ) ;
#5076=CARTESIAN_POINT ( 'NONE',  ( 51.59606816583843170, 11.17458954617364242, 11.97181229448534800 ) ) ;
#5083=CARTESIAN_POINT ( 'NONE',  ( 58.59375000000000711, 11.24264068711927322, 11.99999999999998934 ) ) ;
#5104=CARTESIAN_POINT ( 'NONE',  ( 51.56250000000000711, 5.999999999999996447, 15.00000000000001599 ) ) ;
#5122=CARTESIAN_POINT ( 'NONE',  ( 51.18750000000000711, 9.999999999999978684, 10.99999999999999645 ) ) ;
#5131=CARTESIAN_POINT ( 'NONE',  ( 52.56018183416157541, 7.000000000000000000, 14.93194885905437097 ) ) ;
#5140=CARTESIAN_POINT ( 'NONE',  ( 57.46875000000000711, 6.999999999999992006, 13.75735931288071967 ) ) ;
#5173=CARTESIAN_POINT ( 'NONE',  ( 55.56018183416157541, 5.999999999999996447, 14.93194885905437808 ) ) ;
#5182=CARTESIAN_POINT ( 'NONE',  ( 50.37731816583844591, 7.830560233210212218, 12.92679907967049679 ) ) ;
#5190=CARTESIAN_POINT ( 'NONE',  ( 57.09375000000000711, 11.24264068711927322, 11.99999999999998934 ) ) ;
#5192=CARTESIAN_POINT ( 'NONE',  ( 56.34375000000000711, 8.757359312880723223, 18.00000000000000355 ) ) ;
#5202=CARTESIAN_POINT ( 'NONE',  ( 57.37500000000000000, 7.878679656440349177, 12.87867965644035984 ) ) ;
#5218=CARTESIAN_POINT ( 'NONE',  ( 51.09375000000000000, 11.65685424949236193, 10.99999999999998401 ) ) ;
#5220=FILL_AREA_STYLE ('',( #21613 ) ) ;
#5238=CARTESIAN_POINT ( 'NONE',  ( 52.96875000000000000, 5.999999999999987566, 13.34314575050763452 ) ) ;
#5248=CARTESIAN_POINT ( 'NONE',  ( 58.84143183416158962, 8.275094609562001935, 18.97181229448536044 ) ) ;
#5259=CARTESIAN_POINT ( 'NONE',  ( 55.50000000000000711, 12.12132034355963484, 12.87867965644034740 ) ) ;
#5295=CARTESIAN_POINT ( 'NONE',  ( 54.71643183416158251, 13.97181229448536399, 16.72490539043799629 ) ) ;
#5305=CARTESIAN_POINT ( 'NONE',  ( 52.34606816583843880, 8.825410453826357582, 18.02818770551464667 ) ) ;
#5312=CARTESIAN_POINT ( 'NONE',  ( 53.53125000000000000, 11.24264068711929276, 18.00000000000000355 ) ) ;
#5314=CARTESIAN_POINT ( 'NONE',  ( 58.31250000000000000, 13.00000000000000000, 14.99999999999998757 ) ) ;
#5324=CARTESIAN_POINT ( 'NONE',  ( 55.78125000000000000, 8.757359312880703683, 11.99999999999999822 ) ) ;
#5344=CARTESIAN_POINT ( 'NONE',  ( 58.06481816583843170, 5.999999999999996447, 15.06805114094564502 ) ) ;
#5346=PRESENTATION_STYLE_ASSIGNMENT (( #1740 ) ) ;
#5359=CARTESIAN_POINT ( 'NONE',  ( 56.71875000000000711, 14.00000000000001066, 16.65685424949235482 ) ) ;
#5363=CARTESIAN_POINT ( 'NONE',  ( 52.12500000000000711, 12.82842712474620228, 17.82842712474617386 ) ) ;
#5373=CARTESIAN_POINT ( 'NONE',  ( 53.49768183416157541, 12.16943976678977535, 12.92679907967048614 ) ) ;
#5383=CARTESIAN_POINT ( 'NONE',  ( 59.25000000000000711, 7.878679656440361612, 17.12132034355964549 ) ) ;
#5414=CARTESIAN_POINT ( 'NONE',  ( 52.56018183416157541, 5.999999999999996447, 14.93194885905437808 ) ) ;
#5422=CARTESIAN_POINT ( 'NONE',  ( 54.03356816583844591, 11.31069182806492712, 17.97181229448534623 ) ) ;
#5430=CARTESIAN_POINT ( 'NONE',  ( 51.37500000000000711, 7.878679656440349177, 12.87867965644035984 ) ) ;
#5433=CARTESIAN_POINT ( 'NONE',  ( 55.50000000000000711, 12.12132034355963484, 12.87867965644034740 ) ) ;
#5440=CARTESIAN_POINT ( 'NONE',  ( 52.21875000000002842, 13.00000000000000711, 16.24264068711927322 ) ) ;
#5459=CARTESIAN_POINT ( 'NONE',  ( 51.97106816583844591, 5.971812294485345340, 13.41119689145326710 ) ) ;
#5471=CARTESIAN_POINT ( 'NONE',  ( 54.56250000000000711, 5.999999999999996447, 15.00000000000001599 ) ) ;
#5476=CARTESIAN_POINT ( 'NONE',  ( 52.62731816583844591, 12.87654654797634102, 17.78030770151602979 ) ) ;
#5486=CARTESIAN_POINT ( 'NONE',  ( 54.34143183416158251, 8.275094609562001935, 18.97181229448536044 ) ) ;
#5496=CARTESIAN_POINT ( 'NONE',  ( 53.34375000000000000, 8.757359312880723223, 18.00000000000000711 ) ) ;
#5513=CARTESIAN_POINT ( 'NONE',  ( 60.00000000000000711, 12.82842712474617741, 12.17157287525379239 ) ) ;
#5521=B_SPLINE_CURVE_WITH_KNOTS ( 'NONE', 3,
 ( #7950, #6150, #2771, #10112, #4339, #5047, #3003, #21193, #8898, #6619, #12380, #23480, #16194, #3364, #7094, #12625, #3488, #14172, #15955, #1205, #19645, #10354, #21551, #15849, #19887, #19405, #23237, #8657, #3246, #17751, #13937, #21433, #6847, #23014, #8542, #14290, #14411, #4807, #21307, #1435, #14042, #12139, #10592, #17863, #12505, #17644, #21672, #8776, #23121, #12266, #6734, #16081, #23368, #4929, #19762, #19531 ),
 .UNSPECIFIED., .F., .F.,
 ( 4, 2, 2, 2, 2, 2, 2, 2, 2, 2, 2, 2, 2, 2, 2, 2, 2, 2, 2, 2, 2, 2, 2, 2, 2, 2, 2, 4 ),
 ( 0.000000000000000000, 0.0009277918325622039331, 0.001855583665124407866, 0.002319479581405509399, 0.002783375497686610932, 0.003247271413967717235, 0.003711167330248823972, 0.004638959162811037013, 0.005566750995373249619, 0.006030646911654353320, 0.006262594869794909508, 0.006378568848865185867, 0.006494542827935463093, 0.006552529817470603875, 0.006610516807005745524, 0.006726490786076029689, 0.006958438744216604091, 0.007422334660497751160, 0.008350126493060048768, 0.009277918325622346377, 0.009741814241903491711, 0.01020571015818463531, 0.01113350199074691731, 0.01206129382330919410, 0.01298908565587147089, 0.01345298157215261102, 0.01391687748843375289, 0.01484466932099604008 ),
 .UNSPECIFIED. ) ;
#5526=CARTESIAN_POINT ( 'NONE',  ( 58.09143183416158962, 11.72490539043799984, 11.02818770551463246 ) ) ;
#5535=CARTESIAN_POINT ( 'NONE',  ( 52.53356816583844591, 11.31069182806492712, 17.97181229448534623 ) ) ;
#5543=CARTESIAN_POINT ( 'NONE',  ( 51.93750000000000711, 10.00000000000000711, 17.99999999999999645 ) ) ;
#5545=CARTESIAN_POINT ( 'NONE',  ( 54.46875000000000000, 6.999999999999992895, 13.75735931288071967 ) ) ;
#5554=CARTESIAN_POINT ( 'NONE',  ( 56.81250000000000000, 13.00000000000000000, 14.99999999999998757 ) ) ;
#5575=CARTESIAN_POINT ( 'NONE',  ( 50.84606816583843880, 8.411196891453267099, 19.02818770551464667 ) ) ;
#5592=CARTESIAN_POINT ( 'NONE',  ( 56.43750000000000000, 10.00000000000001776, 18.99999999999999645 ) ) ;
#5598=CARTESIAN_POINT ( 'NONE',  ( 51.68981816583844591, 9.931948859054346102, 10.99999999999999467 ) ) ;
#5606=CARTESIAN_POINT ( 'NONE',  ( 54.62268183416157541, 12.78030770151606177, 17.87654654797631792 ) ) ;
#5646=CARTESIAN_POINT ( 'NONE',  ( 56.87268183416158962, 7.219692298483935566, 12.12345345202367675 ) ) ;
#5654=CARTESIAN_POINT ( 'NONE',  ( 51.50231816583844591, 12.07320092032949610, 12.83056023321021044 ) ) ;
#5661=CARTESIAN_POINT ( 'NONE',  ( 60.24768183416157541, 7.830560233210222876, 17.07320092032950498 ) ) ;
#5665=CARTESIAN_POINT ( 'NONE',  ( 51.56250000000000711, 6.999999999999997335, 15.00000000000000533 ) ) ;
#5673=CARTESIAN_POINT ( 'NONE',  ( 55.87500000000000711, 7.878679656440349177, 12.87867965644035984 ) ) ;
#5693=CARTESIAN_POINT ( 'NONE',  ( 52.53356816583844591, 11.72490539043803004, 18.97181229448534268 ) ) ;
#5710=CARTESIAN_POINT ( 'NONE',  ( 55.59375000000002132, 11.65685424949236015, 10.99999999999998579 ) ) ;
#5715=CARTESIAN_POINT ( 'NONE',  ( 56.18981816583843170, 9.931948859054346102, 10.99999999999999467 ) ) ;
#5727=CARTESIAN_POINT ( 'NONE',  ( 53.12268183416157541, 12.78030770151606177, 17.87654654797631792 ) ) ;
#5774=CARTESIAN_POINT ( 'NONE',  ( 57.56250000000000000, 5.999999999999996447, 15.00000000000001599 ) ) ;
#5781=CARTESIAN_POINT ( 'NONE',  ( 55.21875000000000000, 13.00000000000000711, 16.24264068711927322 ) ) ;
#5787=CARTESIAN_POINT ( 'NONE',  ( 53.62500000000000711, 12.12132034355964727, 17.12132034355963484 ) ) ;
#5798=CARTESIAN_POINT ( 'NONE',  ( 54.84375000000000000, 8.757359312880723223, 18.00000000000000355 ) ) ;
#5813=CARTESIAN_POINT ( 'NONE',  ( 54.59606816583844591, 11.58880310854672935, 10.97181229448534445 ) ) ;
#5828=CARTESIAN_POINT ( 'NONE',  ( 55.03125000000000711, 11.65685424949239923, 18.99999999999998934 ) ) ;
#5832=CARTESIAN_POINT ( 'NONE',  ( 57.50231816583843170, 12.78030770151603868, 12.12345345202365188 ) ) ;
#5841=CARTESIAN_POINT ( 'NONE',  ( 52.93518183416157541, 9.931948859054379852, 18.99999999999999289 ) ) ;
#5849=CARTESIAN_POINT ( 'NONE',  ( 52.78125000000000000, 8.757359312880703683, 11.99999999999999822 ) ) ;
#5889=CARTESIAN_POINT ( 'NONE',  ( 59.53125000000000000, 11.65685424949239923, 18.99999999999998934 ) ) ;
#5900=CARTESIAN_POINT ( 'NONE',  ( 52.87500000000000711, 7.878679656440349177, 12.87867965644035984 ) ) ;
#5906=CARTESIAN_POINT ( 'NONE',  ( 57.24768183416158962, 7.830560233210222876, 17.07320092032950498 ) ) ;
#5915=CARTESIAN_POINT ( 'NONE',  ( 57.99768183416157541, 12.16943976678977535, 12.92679907967048614 ) ) ;
#5934=CARTESIAN_POINT ( 'NONE',  ( 50.93981816583844591, 10.06805114094564857, 19.00000000000000000 ) ) ;
#5953=CARTESIAN_POINT ( 'NONE',  ( 56.56481816583843170, 5.999999999999996447, 15.06805114094564502 ) ) ;
#5964=CARTESIAN_POINT ( 'NONE',  ( 54.81018183416157541, 14.00000000000000000, 15.06805114094561304 ) ) ;
#5971=CARTESIAN_POINT ( 'NONE',  ( 52.40625000000000000, 12.99999999999999645, 13.75735931288070191 ) ) ;
#6007=CARTESIAN_POINT ( 'NONE',  ( 58.40625000000000711, 13.99999999999999289, 13.34314575050759544 ) ) ;
#6015=CARTESIAN_POINT ( 'NONE',  ( 58.68750000000000000, 9.999999999999989342, 11.99999999999999467 ) ) ;
#6022=CARTESIAN_POINT ( 'NONE',  ( 55.09143183416158962, 11.31069182806491291, 12.02818770551463778 ) ) ;
#6035=CARTESIAN_POINT ( 'NONE',  ( 57.15393183416157541, 6.971812294485357775, 16.17458954617365663 ) ) ;
#6052=CARTESIAN_POINT ( 'NONE',  ( 56.93981816583843170, 10.06805114094563791, 17.99999999999999645 ) ) ;
#6079=CARTESIAN_POINT ( 'NONE',  ( 57.84375000000000711, 8.343145750507638070, 19.00000000000000711 ) ) ;
#6128=CARTESIAN_POINT ( 'NONE',  ( 56.53125000000000711, 11.65685424949239923, 18.99999999999998934 ) ) ;
#6141=CARTESIAN_POINT ( 'NONE',  ( 57.84375000000000711, 8.757359312880723223, 18.00000000000000355 ) ) ;
#6149=CARTESIAN_POINT ( 'NONE',  ( 56.87268183416158962, 7.926799079670491466, 12.83056023321021755 ) ) ;
#6150=CARTESIAN_POINT ( 'NONE',  ( 60.00000000000001421, 12.34294812806585462, 13.10030744094656008 ) ) ;
#6159=CARTESIAN_POINT ( 'NONE',  ( 60.71643183416158962, 12.97181229448535689, 16.31069182806490758 ) ) ;
#6180=CARTESIAN_POINT ( 'NONE',  ( 53.18981816583844591, 9.931948859054354983, 11.99999999999999645 ) ) ;
#6194=CARTESIAN_POINT ( 'NONE',  ( 51.46875000000000711, 5.999999999999987566, 13.34314575050763452 ) ) ;
#6204=CARTESIAN_POINT ( 'NONE',  ( 57.00000000000000000, 12.82842712474617741, 12.17157287525379239 ) ) ;
#6207=CARTESIAN_POINT ( 'NONE',  ( 51.00000000000000711, 12.47487373415290612, 12.52512626584706901 ) ) ;
#6261=CARTESIAN_POINT ( 'NONE',  ( 59.31018183416157541, 12.99999999999999822, 15.06805114094562192 ) ) ;
#6274=CARTESIAN_POINT ( 'NONE',  ( 60.15393183416158962, 6.971812294485357775, 16.17458954617365663 ) ) ;
#6295=CARTESIAN_POINT ( 'NONE',  ( 54.78356816583844591, 8.689308171935074654, 12.02818770551464489 ) ) ;
#6323=CARTESIAN_POINT ( 'NONE',  ( 54.75000000000000711, 7.171572875253819923, 17.82842712474619873 ) ) ;
#6376=CARTESIAN_POINT ( 'NONE',  ( 52.50000000000000711, 12.12132034355963484, 12.87867965644034740 ) ) ;
#6381=CARTESIAN_POINT ( 'NONE',  ( 54.99768183416157541, 12.16943976678977535, 12.92679907967048614 ) ) ;
#6389=CARTESIAN_POINT ( 'NONE',  ( 57.62268183416157541, 12.07320092032950676, 17.16943976678977180 ) ) ;
#6400=CARTESIAN_POINT ( 'NONE',  ( 58.25231816583843170, 7.926799079670502124, 17.16943976678978245 ) ) ;
#6416=CARTESIAN_POINT ( 'NONE',  ( 52.72106816583844591, 13.02818770551464489, 16.17458954617363531 ) ) ;
#6429=CARTESIAN_POINT ( 'NONE',  ( 51.84375000000001421, 8.343145750507636293, 19.00000000000000000 ) ) ;
#6442=CARTESIAN_POINT ( 'NONE',  ( 57.37500000000000000, 7.171572875253794166, 12.17157287525381726 ) ) ;
#6506=CARTESIAN_POINT ( 'NONE',  ( 58.09143183416158962, 11.72490539043799984, 11.02818770551463246 ) ) ;
#6518=CARTESIAN_POINT ( 'NONE',  ( 60.81018183416157541, 14.00000000000000000, 15.06805114094561304 ) ) ;
#6527=CARTESIAN_POINT ( 'NONE',  ( 56.09606816583844591, 11.17458954617364242, 11.97181229448534800 ) ) ;
#6533=CARTESIAN_POINT ( 'NONE',  ( 58.87500000000000711, 7.878679656440349177, 12.87867965644035984 ) ) ;
#6538=CARTESIAN_POINT ( 'NONE',  ( 57.03356816583845301, 11.31069182806492712, 17.97181229448534623 ) ) ;
#6539=PRODUCT_DEFINITION ( 'UNKNOWN', '', #13758, #21037 ) ;
#6563=CARTESIAN_POINT ( 'NONE',  ( 55.31250000000000711, 14.00000000000000000, 14.99999999999997691 ) ) ;
#6613=CARTESIAN_POINT ( 'NONE',  ( 51.46875000000000000, 6.999999999999992895, 13.75735931288071967 ) ) ;
#6618=CARTESIAN_POINT ( 'NONE',  ( 53.12268183416157541, 12.07320092032950676, 17.16943976678977180 ) ) ;
#6619=CARTESIAN_POINT ( 'NONE',  ( 60.00000000000004974, 13.00472853162060538, 15.58205920398491173 ) ) ;
#6628=CARTESIAN_POINT ( 'NONE',  ( 52.09143183416158251, 11.31069182806491291, 12.02818770551463778 ) ) ;
#6642=CARTESIAN_POINT ( 'NONE',  ( 57.97106816583845301, 6.971812294485350670, 13.82541045382635403 ) ) ;
#6652=CARTESIAN_POINT ( 'NONE',  ( 59.71875000000000711, 13.00000000000000711, 16.24264068711927322 ) ) ;
#6676=CARTESIAN_POINT ( 'NONE',  ( 52.68750000000000711, 9.999999999999978684, 10.99999999999999645 ) ) ;
#6691=CARTESIAN_POINT ( 'NONE',  ( 54.28125000000000000, 8.343145750507600766, 11.00000000000000533 ) ) ;
#6724=CARTESIAN_POINT ( 'NONE',  ( 52.31250000000000711, 13.00000000000000000, 14.99999999999998757 ) ) ;
#6734=CARTESIAN_POINT ( 'NONE',  ( 60.00000000000001421, 13.67480539368983017, 13.43375491155203960 ) ) ;
#6745=CARTESIAN_POINT ( 'NONE',  ( 53.31018183416157541, 12.99999999999999822, 15.06805114094562192 ) ) ;
#6754=CARTESIAN_POINT ( 'NONE',  ( 50.56481816583844591, 5.999999999999996447, 15.06805114094564502 ) ) ;
#6761=CARTESIAN_POINT ( 'NONE',  ( 58.21875000000000711, 13.00000000000000711, 16.24264068711927322 ) ) ;
#6764=CARTESIAN_POINT ( 'NONE',  ( 50.65856816583843880, 7.028187705514647554, 16.31069182806492179 ) ) ;
#6772=CARTESIAN_POINT ( 'NONE',  ( 58.21875000000000711, 13.00000000000000711, 16.24264068711927322 ) ) ;
#6773=( NAMED_UNIT ( * ) PLANE_ANGLE_UNIT ( ) SI_UNIT ( $, .RADIAN. ) );
#6790=CARTESIAN_POINT ( 'NONE',  ( 55.43981816583843170, 10.06805114094564857, 19.00000000000000000 ) ) ;
#6805=CARTESIAN_POINT ( 'NONE',  ( 59.71875000000000711, 14.00000000000001066, 16.65685424949235482 ) ) ;
#6809=CARTESIAN_POINT ( 'NONE',  ( 53.43750000000000711, 10.00000000000001776, 18.99999999999999645 ) ) ;
#6847=CARTESIAN_POINT ( 'NONE',  ( 60.00000000000000000, 11.22300884646714891, 18.43052338851150651 ) ) ;
#6858=CARTESIAN_POINT ( 'NONE',  ( 53.87268183416157541, 7.926799079670491466, 12.83056023321021755 ) ) ;
#6872=CARTESIAN_POINT ( 'NONE',  ( 50.93981816583844591, 10.06805114094564857, 19.00000000000000000 ) ) ;
#6881=CARTESIAN_POINT ( 'NONE',  ( 56.71875000000000711, 13.00000000000000711, 16.24264068711927322 ) ) ;
#6884=CARTESIAN_POINT ( 'NONE',  ( 56.62500000000000000, 12.12132034355964727, 17.12132034355963484 ) ) ;
#6894=CARTESIAN_POINT ( 'NONE',  ( 58.03125000000000711, 11.24264068711929276, 18.00000000000000355 ) ) ;
#6917=CARTESIAN_POINT ( 'NONE',  ( 56.65856816583844591, 6.028187705514649330, 16.72490539043803182 ) ) ;
#6939=CARTESIAN_POINT ( 'NONE',  ( 58.72106816583844591, 14.02818770551465377, 16.58880310854672757 ) ) ;
#6954=CARTESIAN_POINT ( 'NONE',  ( 55.03125000000000711, 11.24264068711929276, 18.00000000000000000 ) ) ;
#6981=CARTESIAN_POINT ( 'NONE',  ( 52.56018183416157541, 7.000000000000000000, 14.93194885905437097 ) ) ;
#6990=CARTESIAN_POINT ( 'NONE',  ( 54.40856816583843880, 12.97181229448534978, 13.68930817193506755 ) ) ;
#6999=CARTESIAN_POINT ( 'NONE',  ( 58.31250000000000000, 13.00000000000000000, 14.99999999999998757 ) ) ;
#7001=CARTESIAN_POINT ( 'NONE',  ( 58.78125000000000711, 8.757359312880703683, 11.99999999999999822 ) ) ;
#7011=CARTESIAN_POINT ( 'NONE',  ( 58.31250000000000000, 13.00000000000000000, 14.99999999999998757 ) ) ;
#7033=CARTESIAN_POINT ( 'NONE',  ( 57.68981816583843170, 9.931948859054346102, 10.99999999999999467 ) ) ;
#7051=CARTESIAN_POINT ( 'NONE',  ( 58.43981816583843170, 10.06805114094564857, 19.00000000000000000 ) ) ;
#7061=CARTESIAN_POINT ( 'NONE',  ( 60.06018183416157541, 5.999999999999996447, 14.93194885905437808 ) ) ;
#7070=CARTESIAN_POINT ( 'NONE',  ( 59.71875000000000711, 13.00000000000000533, 16.24264068711927322 ) ) ;
#7094=CARTESIAN_POINT ( 'NONE',  ( 60.00000000000004263, 12.51911211317366046, 16.88872345643414263 ) ) ;
#7104=CARTESIAN_POINT ( 'NONE',  ( 53.87268183416157541, 7.219692298483935566, 12.12345345202367675 ) ) ;
#7115=CARTESIAN_POINT ( 'NONE',  ( 50.00231816583843170, 12.07320092032949610, 12.83056023321021044 ) ) ;
#7122=CARTESIAN_POINT ( 'NONE',  ( 53.06250000000000711, 6.999999999999997335, 15.00000000000000533 ) ) ;
#7125=CARTESIAN_POINT ( 'NONE',  ( 58.40625000000000711, 12.99999999999999645, 13.75735931288070191 ) ) ;
#7133=CARTESIAN_POINT ( 'NONE',  ( 52.87500000000000711, 7.878679656440349177, 12.87867965644035984 ) ) ;
#7152=CARTESIAN_POINT ( 'NONE',  ( 58.25231816583843170, 7.219692298483957771, 17.87654654797633924 ) ) ;
#7168=CARTESIAN_POINT ( 'NONE',  ( 57.09375000000000711, 11.65685424949236015, 10.99999999999998579 ) ) ;
#7173=CARTESIAN_POINT ( 'NONE',  ( 52.21875000000002842, 14.00000000000000888, 16.65685424949235482 ) ) ;
#7185=CARTESIAN_POINT ( 'NONE',  ( 59.02893183416158251, 11.58880310854676132, 19.02818770551463956 ) ) ;
#7194=CARTESIAN_POINT ( 'NONE',  ( 54.37500000000000711, 7.878679656440349177, 12.87867965644035984 ) ) ;
#7211=CIRCLE ( 'NONE', #20558, 0.5000000000000006661 ) ;
#7230=CARTESIAN_POINT ( 'NONE',  ( 52.65393183416158251, 5.971812294485358663, 16.58880310854675599 ) ) ;
#7238=CARTESIAN_POINT ( 'NONE',  ( 54.31481816583844591, 12.99999999999999822, 14.93194885905435676 ) ) ;
#7246=CARTESIAN_POINT ( 'NONE',  ( 52.31250000000000711, 13.00000000000000000, 14.99999999999998757 ) ) ;
#7248=CARTESIAN_POINT ( 'NONE',  ( 52.96875000000000000, 6.999999999999992895, 13.75735931288071967 ) ) ;
#7257=CARTESIAN_POINT ( 'NONE',  ( 52.68750000000000711, 9.999999999999989342, 11.99999999999999467 ) ) ;
#7280=CARTESIAN_POINT ( 'NONE',  ( 53.18981816583844591, 9.931948859054346102, 10.99999999999999467 ) ) ;
#7296=CARTESIAN_POINT ( 'NONE',  ( 57.00000000000000000, 12.82842712474617741, 12.17157287525379239 ) ) ;
#7301=CARTESIAN_POINT ( 'NONE',  ( 55.06481816583844591, 5.999999999999996447, 15.06805114094564502 ) ) ;
#7312=CARTESIAN_POINT ( 'NONE',  ( 52.84143183416158251, 8.689308171935088865, 17.97181229448535689 ) ) ;
#7318=AXIS2_PLACEMENT_3D ( 'NONE', #3111, #10686, #17843 ) ;
#7321=CARTESIAN_POINT ( 'NONE',  ( 56.43750000000000000, 10.00000000000000711, 17.99999999999999645 ) ) ;
#7354=CARTESIAN_POINT ( 'NONE',  ( 54.99768183416157541, 12.87654654797631792, 12.21969229848393113 ) ) ;
#7361=CARTESIAN_POINT ( 'NONE',  ( 53.65856816583844591, 7.028187705514647554, 16.31069182806492179 ) ) ;
#7367=CARTESIAN_POINT ( 'NONE',  ( 55.40625000000000000, 12.99999999999999645, 13.75735931288070191 ) ) ;
#7370=CARTESIAN_POINT ( 'NONE',  ( 56.25000000000000711, 7.878679656440361612, 17.12132034355964549 ) ) ;
#7379=CARTESIAN_POINT ( 'NONE',  ( 57.00000000000000000, 12.12132034355963484, 12.87867965644034740 ) ) ;
#7394=CARTESIAN_POINT ( 'NONE',  ( 53.09606816583843170, 11.58880310854672935, 10.97181229448534445 ) ) ;
#7409=CARTESIAN_POINT ( 'NONE',  ( 54.93750000000000711, 10.00000000000001776, 18.99999999999999645 ) ) ;
#7414=CARTESIAN_POINT ( 'NONE',  ( 57.03356816583845301, 11.72490539043803004, 18.97181229448534268 ) ) ;
#7423=CARTESIAN_POINT ( 'NONE',  ( 59.34375000000000711, 8.343145750507638070, 19.00000000000000711 ) ) ;
#7461=CARTESIAN_POINT ( 'NONE',  ( 54.90393183416157541, 14.02818770551463956, 13.41119689145323335 ) ) ;
#7469=CARTESIAN_POINT ( 'NONE',  ( 50.75231816583844591, 7.926799079670502124, 17.16943976678978245 ) ) ;
#7479=CARTESIAN_POINT ( 'NONE',  ( 53.81250000000000711, 13.00000000000000000, 14.99999999999998757 ) ) ;
#7481=CARTESIAN_POINT ( 'NONE',  ( 51.84375000000001421, 8.757359312880723223, 18.00000000000000355 ) ) ;
#7488=CARTESIAN_POINT ( 'NONE',  ( 56.90625000000000711, 12.99999999999999645, 13.75735931288070191 ) ) ;
#7509=CARTESIAN_POINT ( 'NONE',  ( 52.34606816583843880, 8.411196891453267099, 19.02818770551464667 ) ) ;
#7522=CARTESIAN_POINT ( 'NONE',  ( 57.37500000000000000, 7.171572875253794166, 12.17157287525381726 ) ) ;
#7526=CARTESIAN_POINT ( 'NONE',  ( 53.47106816583843880, 5.971812294485345340, 13.41119689145326710 ) ) ;
#7535=CARTESIAN_POINT ( 'NONE',  ( 55.65393183416158251, 5.971812294485358663, 16.58880310854675599 ) ) ;
#7579=CARTESIAN_POINT ( 'NONE',  ( 57.28125000000000711, 8.343145750507600766, 11.00000000000000533 ) ) ;
#7588=CARTESIAN_POINT ( 'NONE',  ( 54.37500000000000711, 7.878679656440349177, 12.87867965644035984 ) ) ;
#7593=CARTESIAN_POINT ( 'NONE',  ( 59.87268183416157541, 7.926799079670491466, 12.83056023321021755 ) ) ;
#7596=EDGE_CURVE ( 'NONE', #10540, #1478, #13233, .T. ) ;
#7608=CARTESIAN_POINT ( 'NONE',  ( 55.59375000000000711, 11.24264068711927322, 11.99999999999998934 ) ) ;
#7627=CARTESIAN_POINT ( 'NONE',  ( 58.81481816583843170, 12.99999999999999822, 14.93194885905435676 ) ) ;
#7646=CARTESIAN_POINT ( 'NONE',  ( 53.62500000000000711, 12.82842712474620228, 17.82842712474617386 ) ) ;
#7651=CARTESIAN_POINT ( 'NONE',  ( 54.12731816583844591, 12.87654654797634102, 17.78030770151602979 ) ) ;
#7657=CARTESIAN_POINT ( 'NONE',  ( 54.15393183416158251, 5.971812294485358663, 16.58880310854675599 ) ) ;
#7705=CARTESIAN_POINT ( 'NONE',  ( 58.03125000000000711, 11.65685424949239923, 18.99999999999998934 ) ) ;
#7714=CARTESIAN_POINT ( 'NONE',  ( 53.06250000000000711, 6.999999999999997335, 15.00000000000000533 ) ) ;
#7722=CARTESIAN_POINT ( 'NONE',  ( 57.99768183416157541, 12.16943976678977535, 12.92679907967048614 ) ) ;
#7724=CARTESIAN_POINT ( 'NONE',  ( 52.40625000000000000, 12.99999999999999645, 13.75735931288070191 ) ) ;
#7732=CARTESIAN_POINT ( 'NONE',  ( 57.52893183416158962, 11.17458954617365663, 18.02818770551464311 ) ) ;
#7748=CARTESIAN_POINT ( 'NONE',  ( 51.68981816583844591, 9.931948859054346102, 10.99999999999999467 ) ) ;
#7760=CARTESIAN_POINT ( 'NONE',  ( 51.18750000000000711, 9.999999999999978684, 10.99999999999999645 ) ) ;
#7764=CARTESIAN_POINT ( 'NONE',  ( 55.53356816583845301, 11.72490539043803004, 18.97181229448534268 ) ) ;
#7770=ADVANCED_FACE ( 'NONE', ( #3294 ), #14336, .T. ) ;
#7775=CARTESIAN_POINT ( 'NONE',  ( 59.62500000000000711, 12.82842712474620228, 17.82842712474617386 ) ) ;
#7782=CARTESIAN_POINT ( 'NONE',  ( 54.09375000000000711, 11.24264068711927322, 11.99999999999998934 ) ) ;
#7816=CARTESIAN_POINT ( 'NONE',  ( 56.25000000000000711, 7.171572875253819923, 17.82842712474619873 ) ) ;
#7824=CARTESIAN_POINT ( 'NONE',  ( 57.75000000000000000, 7.878679656440361612, 17.12132034355964549 ) ) ;
#7830=CARTESIAN_POINT ( 'NONE',  ( 55.84143183416158251, 8.689308171935088865, 17.97181229448535689 ) ) ;
#7839=CARTESIAN_POINT ( 'NONE',  ( 55.56018183416157541, 7.000000000000000000, 14.93194885905437097 ) ) ;
#7856=CARTESIAN_POINT ( 'NONE',  ( 55.81481816583843170, 12.99999999999999822, 14.93194885905435676 ) ) ;
#7885=CARTESIAN_POINT ( 'NONE',  ( 55.84143183416158251, 8.275094609562001935, 18.97181229448536044 ) ) ;
#7895=CARTESIAN_POINT ( 'NONE',  ( 53.06250000000000711, 6.999999999999997335, 15.00000000000000533 ) ) ;
#7927=ORIENTED_EDGE ( 'NONE', *, *, #8075, .T. ) ;
#7931=CARTESIAN_POINT ( 'NONE',  ( 56.71875000000000711, 14.00000000000000888, 16.65685424949235482 ) ) ;
#7941=CARTESIAN_POINT ( 'NONE',  ( 58.59375000000000711, 11.24264068711927322, 11.99999999999998934 ) ) ;
#7949=CARTESIAN_POINT ( 'NONE',  ( 54.06018183416157541, 7.000000000000000000, 14.93194885905437097 ) ) ;
#7950=CARTESIAN_POINT ( 'NONE',  ( 60.00000000000000711, 12.12132034355963484, 12.87867965644034740 ) ) ;
#7960=CARTESIAN_POINT ( 'NONE',  ( 57.24768183416158962, 7.830560233210222876, 17.07320092032950498 ) ) ;
#7982=CARTESIAN_POINT ( 'NONE',  ( 55.62731816583843170, 12.16943976678978601, 17.07320092032949432 ) ) ;
#7985=DIRECTION ( 'NONE',  ( 0.06805114094563521898, -0.7054675904022857935, -0.7054675904022735811 ) ) ;
#8009=CARTESIAN_POINT ( 'NONE',  ( 55.59375000000000711, 11.65685424949236193, 10.99999999999998401 ) ) ;
#8011=DIRECTION ( 'NONE',  ( 0.06805114094563521898, -0.7054675904022857935, -0.7054675904022735811 ) ) ;
#8030=STYLED_ITEM ( 'NONE', ( #17564 ), #23619 ) ;
#8060=CARTESIAN_POINT ( 'NONE',  ( 58.12500000000000000, 12.82842712474620228, 17.82842712474617386 ) ) ;
#8070=CARTESIAN_POINT ( 'NONE',  ( 54.84375000000000000, 8.757359312880723223, 18.00000000000000355 ) ) ;
#8075=EDGE_CURVE ( 'NONE', #10540, #16693, #7211, .T. ) ;
#8080=CARTESIAN_POINT ( 'NONE',  ( 57.15393183416157541, 6.971812294485357775, 16.17458954617365663 ) ) ;
#8091=CARTESIAN_POINT ( 'NONE',  ( 60.62268183416157541, 12.07320092032950676, 17.16943976678977180 ) ) ;
#8111=CARTESIAN_POINT ( 'NONE',  ( 56.37731816583843170, 7.830560233210212218, 12.92679907967049679 ) ) ;
#8128=UNCERTAINTY_MEASURE_WITH_UNIT (LENGTH_MEASURE( 1.000000000000000082E-05 ), #8580, 'distance_accuracy_value', 'NONE');
#8134=CARTESIAN_POINT ( 'NONE',  ( 55.21875000000000000, 14.00000000000000888, 16.65685424949235482 ) ) ;
#8188=CARTESIAN_POINT ( 'NONE',  ( 54.81018183416157541, 12.99999999999999822, 15.06805114094562192 ) ) ;
#8199=CARTESIAN_POINT ( 'NONE',  ( 59.59143183416158962, 11.31069182806491291, 12.02818770551463778 ) ) ;
#8202=ORIENTED_EDGE ( 'NONE', *, *, #17689, .F. ) ;
#8209=CARTESIAN_POINT ( 'NONE',  ( 56.93981816583843170, 10.06805114094563791, 17.99999999999999645 ) ) ;
#8219=CARTESIAN_POINT ( 'NONE',  ( 57.22106816583844591, 13.02818770551464489, 16.17458954617363531 ) ) ;
#8247=CARTESIAN_POINT ( 'NONE',  ( 54.18750000000000711, 9.999999999999978684, 10.99999999999999645 ) ) ;
#8301=CARTESIAN_POINT ( 'NONE',  ( 59.87268183416157541, 7.219692298483935566, 12.12345345202367675 ) ) ;
#8310=CARTESIAN_POINT ( 'NONE',  ( 53.68518183416157541, 10.06805114094562548, 11.99999999999999645 ) ) ;
#8318=CARTESIAN_POINT ( 'NONE',  ( 58.53356816583845301, 11.31069182806492712, 17.97181229448534623 ) ) ;
#8331=FACE_OUTER_BOUND ( 'NONE', #18190, .T. ) ;
#8336=CARTESIAN_POINT ( 'NONE',  ( 52.62731816583844591, 12.16943976678978601, 17.07320092032949432 ) ) ;
#8345=SURFACE_STYLE_FILL_AREA ( #13740 ) ;
#8364=CARTESIAN_POINT ( 'NONE',  ( 56.15625000000002132, 6.000000000000004441, 16.65685424949239390 ) ) ;
#8431=CARTESIAN_POINT ( 'NONE',  ( 57.71643183416158251, 13.97181229448536399, 16.72490539043799629 ) ) ;
#8443=CARTESIAN_POINT ( 'NONE',  ( 60.62268183416157541, 12.78030770151606177, 17.87654654797631792 ) ) ;
#8454=CARTESIAN_POINT ( 'NONE',  ( 50.47106816583844591, 5.971812294485345340, 13.41119689145326710 ) ) ;
#8460=CARTESIAN_POINT ( 'NONE',  ( 58.68750000000000000, 9.999999999999989342, 11.99999999999999467 ) ) ;
#8465=CARTESIAN_POINT ( 'NONE',  ( 50.00231816583843170, 12.07320092032949610, 12.83056023321021044 ) ) ;
#8474=CARTESIAN_POINT ( 'NONE',  ( 59.53125000000000000, 11.24264068711929276, 18.00000000000000355 ) ) ;
#8489=CARTESIAN_POINT ( 'NONE',  ( 58.21875000000000711, 14.00000000000000888, 16.65685424949235482 ) ) ;
#8542=CARTESIAN_POINT ( 'NONE',  ( 60.00000000000002842, 11.59862743136960717, 18.35022190915677243 ) ) ;
#8551=CARTESIAN_POINT ( 'NONE',  ( 54.90393183416157541, 13.02818770551463778, 13.82541045382633982 ) ) ;
#8561=CARTESIAN_POINT ( 'NONE',  ( 56.28356816583844591, 8.689308171935074654, 12.02818770551464489 ) ) ;
#8567=CARTESIAN_POINT ( 'NONE',  ( 59.06250000000000711, 6.999999999999997335, 15.00000000000000533 ) ) ;
#8570=CARTESIAN_POINT ( 'NONE',  ( 58.21875000000000711, 13.00000000000000711, 16.24264068711927322 ) ) ;
#8579=CARTESIAN_POINT ( 'NONE',  ( 58.50000000000000000, 12.12132034355963484, 12.87867965644034740 ) ) ;
#8580=( LENGTH_UNIT ( ) NAMED_UNIT ( * ) SI_UNIT ( .MILLI., .METRE. ) );
#8596=CARTESIAN_POINT ( 'NONE',  ( 57.59606816583843880, 11.58880310854672935, 10.97181229448534445 ) ) ;
#8614=CARTESIAN_POINT ( 'NONE',  ( 58.62731816583843170, 12.87654654797634102, 17.78030770151602979 ) ) ;
#8632=CARTESIAN_POINT ( 'NONE',  ( 55.31250000000000711, 13.00000000000000000, 14.99999999999998757 ) ) ;
#8657=CARTESIAN_POINT ( 'NONE',  ( 59.99999999999998579, 10.91440514551900698, 18.40918491980847804 ) ) ;
#8668=CARTESIAN_POINT ( 'NONE',  ( 54.99768183416157541, 12.16943976678977535, 12.92679907967048614 ) ) ;
#8676=VERTEX_POINT ( 'NONE', #23657 ) ;
#8677=CARTESIAN_POINT ( 'NONE',  ( 51.40856816583843880, 13.97181229448534978, 13.27509460956196641 ) ) ;
#8684=CARTESIAN_POINT ( 'NONE',  ( 57.75000000000000000, 7.878679656440361612, 17.12132034355964549 ) ) ;
#8686=CARTESIAN_POINT ( 'NONE',  ( 51.12731816583844591, 12.16943976678978601, 17.07320092032949432 ) ) ;
#8713=CARTESIAN_POINT ( 'NONE',  ( 52.96875000000000000, 5.999999999999987566, 13.34314575050763452 ) ) ;
#8727=CARTESIAN_POINT ( 'NONE',  ( 59.25000000000000711, 7.171572875253819923, 17.82842712474619873 ) ) ;
#8732=CARTESIAN_POINT ( 'NONE',  ( 57.59606816583843880, 11.58880310854672935, 10.97181229448534445 ) ) ;
#8750=CARTESIAN_POINT ( 'NONE',  ( 56.15625000000001421, 7.000000000000002665, 16.24264068711929099 ) ) ;
#8776=CARTESIAN_POINT ( 'NONE',  ( 60.00000000000001421, 13.93055609735682054, 14.31316200167426267 ) ) ;
#8786=CARTESIAN_POINT ( 'NONE',  ( 54.06018183416157541, 7.000000000000000000, 14.93194885905437097 ) ) ;
#8802=CARTESIAN_POINT ( 'NONE',  ( 50.65856816583843880, 7.028187705514647554, 16.31069182806492179 ) ) ;
#8812=CARTESIAN_POINT ( 'NONE',  ( 59.62500000000000711, 12.12132034355964727, 17.12132034355963484 ) ) ;
#8815=CARTESIAN_POINT ( 'NONE',  ( 56.90625000000000711, 12.99999999999999645, 13.75735931288070191 ) ) ;
#8824=CARTESIAN_POINT ( 'NONE',  ( 59.06250000000000711, 6.999999999999997335, 15.00000000000000533 ) ) ;
#8846=CARTESIAN_POINT ( 'NONE',  ( 58.34606816583844591, 8.411196891453267099, 19.02818770551464667 ) ) ;
#8862=CARTESIAN_POINT ( 'NONE',  ( 53.71875000000002132, 14.00000000000000888, 16.65685424949235482 ) ) ;
#8873=CARTESIAN_POINT ( 'NONE',  ( 57.34143183416159673, 8.275094609562001935, 18.97181229448536044 ) ) ;
#8881=CARTESIAN_POINT ( 'NONE',  ( 59.06250000000000711, 6.999999999999997335, 15.00000000000000533 ) ) ;
#8898=CARTESIAN_POINT ( 'NONE',  ( 60.00000000000004263, 13.03655146502352480, 15.27384441607152965 ) ) ;
#8910=CARTESIAN_POINT ( 'NONE',  ( 58.37268183416157541, 7.219692298483935566, 12.12345345202367675 ) ) ;
#8922=CARTESIAN_POINT ( 'NONE',  ( 54.50231816583843170, 12.07320092032949610, 12.83056023321021044 ) ) ;
#8928=CARTESIAN_POINT ( 'NONE',  ( 52.78125000000000711, 8.757359312880703683, 11.99999999999999822 ) ) ;
#8931=CARTESIAN_POINT ( 'NONE',  ( 51.87731816583844591, 7.830560233210212218, 12.92679907967049679 ) ) ;
#8941=CARTESIAN_POINT ( 'NONE',  ( 54.18750000000000711, 9.999999999999989342, 11.99999999999999467 ) ) ;
#8963=CARTESIAN_POINT ( 'NONE',  ( 52.12500000000000711, 12.82842712474620228, 17.82842712474617386 ) ) ;
#8982=CARTESIAN_POINT ( 'NONE',  ( 58.96875000000000711, 5.999999999999987566, 13.34314575050763452 ) ) ;
#8986=CARTESIAN_POINT ( 'NONE',  ( 52.87500000000000711, 7.171572875253794166, 12.17157287525381726 ) ) ;
#8994=CARTESIAN_POINT ( 'NONE',  ( 52.65393183416158251, 6.971812294485357775, 16.17458954617365663 ) ) ;
#9000=CARTESIAN_POINT ( 'NONE',  ( 54.56250000000000711, 6.999999999999997335, 15.00000000000000533 ) ) ;
#9032=CARTESIAN_POINT ( 'NONE',  ( 52.84143183416158251, 8.275094609562001935, 18.97181229448536044 ) ) ;
#9039=CARTESIAN_POINT ( 'NONE',  ( 58.78125000000000711, 8.757359312880703683, 11.99999999999999822 ) ) ;
#9047=CARTESIAN_POINT ( 'NONE',  ( 52.68750000000000711, 9.999999999999989342, 11.99999999999999467 ) ) ;
#9049=CARTESIAN_POINT ( 'NONE',  ( 55.03125000000000000, 11.24264068711929276, 18.00000000000000355 ) ) ;
#9056=CARTESIAN_POINT ( 'NONE',  ( 56.06250000000000000, 6.999999999999997335, 15.00000000000000533 ) ) ;
#9076=CARTESIAN_POINT ( 'NONE',  ( 53.65856816583844591, 6.028187705514649330, 16.72490539043803182 ) ) ;
#9089=CARTESIAN_POINT ( 'NONE',  ( 55.78125000000000711, 8.343145750507600766, 11.00000000000000355 ) ) ;
#9094=CARTESIAN_POINT ( 'NONE',  ( 57.40856816583844591, 13.97181229448534978, 13.27509460956196641 ) ) ;
#9107=CARTESIAN_POINT ( 'NONE',  ( 56.96643183416158251, 6.028187705514633343, 13.27509460956200016 ) ) ;
#9116=CARTESIAN_POINT ( 'NONE',  ( 58.59375000000000711, 11.24264068711927322, 11.99999999999998934 ) ) ;
#9153=CARTESIAN_POINT ( 'NONE',  ( 57.62268183416157541, 12.78030770151606177, 17.87654654797631792 ) ) ;
#9162=CARTESIAN_POINT ( 'NONE',  ( 52.81481816583844591, 12.99999999999999822, 14.93194885905435676 ) ) ;
#9170=CARTESIAN_POINT ( 'NONE',  ( 53.43750000000000711, 10.00000000000000711, 17.99999999999999645 ) ) ;
#9173=CARTESIAN_POINT ( 'NONE',  ( 53.25000000000000711, 7.878679656440361612, 17.12132034355964549 ) ) ;
#9182=CARTESIAN_POINT ( 'NONE',  ( 51.84375000000001421, 8.757359312880723223, 18.00000000000000355 ) ) ;
#9200=CARTESIAN_POINT ( 'NONE',  ( 51.03356816583844591, 11.72490539043803004, 18.97181229448534268 ) ) ;
#9215=CARTESIAN_POINT ( 'NONE',  ( 56.25000000000000711, 7.171572875253819923, 17.82842712474619873 ) ) ;
#9220=CARTESIAN_POINT ( 'NONE',  ( 55.90856816583843880, 13.97181229448534978, 13.27509460956196641 ) ) ;
#9228=CARTESIAN_POINT ( 'NONE',  ( 56.31018183416157541, 14.00000000000000000, 15.06805114094561304 ) ) ;
#9237=CARTESIAN_POINT ( 'NONE',  ( 51.28125000000000000, 8.757359312880703683, 11.99999999999999822 ) ) ;
#9269=CARTESIAN_POINT ( 'NONE',  ( 56.02893183416158962, 11.58880310854676132, 19.02818770551463956 ) ) ;
#9277=CARTESIAN_POINT ( 'NONE',  ( 52.15856816583843880, 7.028187705514647554, 16.31069182806492179 ) ) ;
#9282=CARTESIAN_POINT ( 'NONE',  ( 60.71643183416158962, 12.97181229448535689, 16.31069182806490758 ) ) ;
#9284=CARTESIAN_POINT ( 'NONE',  ( 54.18750000000000711, 9.999999999999989342, 11.99999999999999467 ) ) ;
#9291=CARTESIAN_POINT ( 'NONE',  ( 52.03124999999999289, 11.24264068711929276, 18.00000000000000355 ) ) ;
#9308=CARTESIAN_POINT ( 'NONE',  ( 50.47106816583844591, 5.971812294485345340, 13.41119689145326710 ) ) ;
#9321=CARTESIAN_POINT ( 'NONE',  ( 58.40625000000000711, 13.99999999999999289, 13.34314575050759544 ) ) ;
#9325=CARTESIAN_POINT ( 'NONE',  ( 54.40856816583843880, 13.97181229448534978, 13.27509460956196641 ) ) ;
#9336=CARTESIAN_POINT ( 'NONE',  ( 59.06250000000000711, 5.999999999999996447, 15.00000000000001599 ) ) ;
#9379=CARTESIAN_POINT ( 'NONE',  ( 57.81018183416157541, 14.00000000000000000, 15.06805114094561304 ) ) ;
#9387=CARTESIAN_POINT ( 'NONE',  ( 53.90625000000000000, 12.99999999999999645, 13.75735931288070191 ) ) ;
#9395=CARTESIAN_POINT ( 'NONE',  ( 60.90393183416158962, 13.02818770551463778, 13.82541045382633982 ) ) ;
#9406=CARTESIAN_POINT ( 'NONE',  ( 56.43750000000000000, 10.00000000000000711, 17.99999999999999645 ) ) ;
#9409=CIRCLE ( 'NONE', #11335, 0.5000000000000006661 ) ;
#9425=CARTESIAN_POINT ( 'NONE',  ( 53.47106816583843880, 5.971812294485345340, 13.41119689145326710 ) ) ;
#9437=CARTESIAN_POINT ( 'NONE',  ( 54.75000000000000711, 7.171572875253819923, 17.82842712474619873 ) ) ;
#9441=CARTESIAN_POINT ( 'NONE',  ( 54.87731816583843170, 7.123453452023657206, 12.21969229848395599 ) ) ;
#9449=CARTESIAN_POINT ( 'NONE',  ( 54.43518183416157541, 9.931948859054379852, 18.99999999999999289 ) ) ;
#9457=CARTESIAN_POINT ( 'NONE',  ( 52.12500000000000711, 12.12132034355964727, 17.12132034355963484 ) ) ;
#9493=CARTESIAN_POINT ( 'NONE',  ( 56.90625000000000711, 13.99999999999999289, 13.34314575050759544 ) ) ;
#9505=CARTESIAN_POINT ( 'NONE',  ( 55.68750000000000000, 9.999999999999989342, 11.99999999999999467 ) ) ;
#9513=CARTESIAN_POINT ( 'NONE',  ( 56.59143183416158962, 11.31069182806491291, 12.02818770551463778 ) ) ;
#9518=CARTESIAN_POINT ( 'NONE',  ( 55.12500000000000711, 12.12132034355964727, 17.12132034355963484 ) ) ;
#9527=CARTESIAN_POINT ( 'NONE',  ( 57.06018183416157541, 7.000000000000000000, 14.93194885905437097 ) ) ;
#9539=EDGE_CURVE ( 'NONE', #10540, #16693, #12814, .T. ) ;
#9547=CARTESIAN_POINT ( 'NONE',  ( 54.87731816583843170, 7.123453452023657206, 12.21969229848395599 ) ) ;
#9552=COLOUR_RGB ( '', 0.31764706, 0.68627451, 0.89019608) ;
#9565=CARTESIAN_POINT ( 'NONE',  ( 51.28125000000000000, 8.343145750507600766, 11.00000000000000355 ) ) ;
#9572=CARTESIAN_POINT ( 'NONE',  ( 55.72106816583844591, 14.02818770551465377, 16.58880310854672757 ) ) ;
#9580=CARTESIAN_POINT ( 'NONE',  ( 59.90625000000000711, 13.99999999999999289, 13.34314575050759544 ) ) ;
#9589=CARTESIAN_POINT ( 'NONE',  ( 52.50000000000000711, 12.12132034355963484, 12.87867965644034740 ) ) ;
#9625=CARTESIAN_POINT ( 'NONE',  ( 56.34375000000000711, 8.343145750507638070, 19.00000000000000711 ) ) ;
#9634=CARTESIAN_POINT ( 'NONE',  ( 56.90625000000000711, 12.99999999999999645, 13.75735931288070191 ) ) ;
#9640=CARTESIAN_POINT ( 'NONE',  ( 58.74768183416157541, 7.830560233210222876, 17.07320092032950498 ) ) ;
#9650=CARTESIAN_POINT ( 'NONE',  ( 57.81018183416157541, 12.99999999999999822, 15.06805114094562192 ) ) ;
#9667=CARTESIAN_POINT ( 'NONE',  ( 56.18981816583843170, 9.931948859054354983, 11.99999999999999645 ) ) ;
#9680=CARTESIAN_POINT ( 'NONE',  ( 51.56250000000000711, 5.999999999999996447, 15.00000000000001599 ) ) ;
#9691=CARTESIAN_POINT ( 'NONE',  ( 53.49768183416157541, 12.87654654797631792, 12.21969229848393113 ) ) ;
#9735=CARTESIAN_POINT ( 'NONE',  ( 55.87500000000000711, 7.171572875253794166, 12.17157287525381726 ) ) ;
#9744=CARTESIAN_POINT ( 'NONE',  ( 56.81250000000000000, 13.00000000000000000, 14.99999999999998757 ) ) ;
#9749=CARTESIAN_POINT ( 'NONE',  ( 54.43518183416157541, 9.931948859054372747, 17.99999999999999645 ) ) ;
#9758=CARTESIAN_POINT ( 'NONE',  ( 60.24768183416157541, 7.830560233210222876, 17.07320092032950498 ) ) ;
#9779=CARTESIAN_POINT ( 'NONE',  ( 54.87731816583843170, 7.830560233210212218, 12.92679907967049679 ) ) ;
#9795=CARTESIAN_POINT ( 'NONE',  ( 52.96875000000000000, 5.999999999999987566, 13.34314575050763452 ) ) ;
#9807=CARTESIAN_POINT ( 'NONE',  ( 58.50000000000000000, 12.82842712474617741, 12.17157287525379239 ) ) ;
#9852=CARTESIAN_POINT ( 'NONE',  ( 59.43750000000000711, 10.00000000000001776, 18.99999999999999645 ) ) ;
#9862=CARTESIAN_POINT ( 'NONE',  ( 56.06250000000000000, 6.999999999999997335, 15.00000000000000533 ) ) ;
#9870=CARTESIAN_POINT ( 'NONE',  ( 59.12268183416157541, 12.07320092032950676, 17.16943976678977180 ) ) ;
#9884=CARTESIAN_POINT ( 'NONE',  ( 55.84143183416158251, 8.689308171935088865, 17.97181229448535689 ) ) ;
#9905=CARTESIAN_POINT ( 'NONE',  ( 56.28356816583844591, 8.689308171935074654, 12.02818770551464489 ) ) ;
#9921=CARTESIAN_POINT ( 'NONE',  ( 51.37500000000000711, 7.171572875253794166, 12.17157287525381726 ) ) ;
#9932=CARTESIAN_POINT ( 'NONE',  ( 55.87500000000000711, 7.171572875253794166, 12.17157287525381726 ) ) ;
#9953=( GEOMETRIC_REPRESENTATION_CONTEXT ( 3 ) GLOBAL_UNCERTAINTY_ASSIGNED_CONTEXT ( ( #8128 ) ) GLOBAL_UNIT_ASSIGNED_CONTEXT ( ( #8580, #17790, #16000 ) ) REPRESENTATION_CONTEXT ( 'NONE', 'WORKASPACE' ) );
#9999=CARTESIAN_POINT ( 'NONE',  ( 55.93518183416157541, 9.931948859054372747, 17.99999999999999645 ) ) ;
#10011=CARTESIAN_POINT ( 'NONE',  ( 60.06018183416157541, 7.000000000000000000, 14.93194885905437097 ) ) ;
#10021=CARTESIAN_POINT ( 'NONE',  ( 56.65856816583844591, 7.028187705514647554, 16.31069182806492179 ) ) ;
#10031=CARTESIAN_POINT ( 'NONE',  ( 53.00231816583844591, 12.07320092032949610, 12.83056023321021044 ) ) ;
#10046=CARTESIAN_POINT ( 'NONE',  ( 53.06250000000000711, 5.999999999999996447, 15.00000000000001599 ) ) ;
#10054=CARTESIAN_POINT ( 'NONE',  ( 58.12500000000000000, 12.82842712474620228, 17.82842712474617386 ) ) ;
#10111=CARTESIAN_POINT ( 'NONE',  ( 60.90393183416158962, 14.02818770551463956, 13.41119689145323335 ) ) ;
#10112=CARTESIAN_POINT ( 'NONE',  ( 59.99999999999999289, 12.81859298856320528, 13.90091681563048631 ) ) ;
#10120=CARTESIAN_POINT ( 'NONE',  ( 58.84143183416158962, 8.275094609562001935, 18.97181229448536044 ) ) ;
#10133=CARTESIAN_POINT ( 'NONE',  ( 58.62731816583843170, 12.16943976678978601, 17.07320092032949432 ) ) ;
#10145=CARTESIAN_POINT ( 'NONE',  ( 54.68981816583844591, 9.931948859054354983, 11.99999999999999645 ) ) ;
#10174=CARTESIAN_POINT ( 'NONE',  ( 55.40625000000000000, 13.99999999999999289, 13.34314575050759544 ) ) ;
#10226=SHAPE_REPRESENTATION ( 'End Stop Bumper spring', ( #7318 ), #9953 ) ;
#10228=CARTESIAN_POINT ( 'NONE',  ( 52.27893183416158251, 8.825410453826341595, 11.97181229448535511 ) ) ;
#10241=CARTESIAN_POINT ( 'NONE',  ( 53.77893183416158251, 8.825410453826341595, 11.97181229448535511 ) ) ;
#10250=CARTESIAN_POINT ( 'NONE',  ( 55.90856816583843880, 12.97181229448534978, 13.68930817193506755 ) ) ;
#10263=CARTESIAN_POINT ( 'NONE',  ( 58.50000000000000000, 12.12132034355963484, 12.87867965644034740 ) ) ;
#10273=CARTESIAN_POINT ( 'NONE',  ( 60.00000000000000711, 12.12132034355963484, 12.87867965644034740 ) ) ;
#10291=CARTESIAN_POINT ( 'NONE',  ( 53.62500000000000711, 12.82842712474620228, 17.82842712474617386 ) ) ;
#10354=CARTESIAN_POINT ( 'NONE',  ( 59.99999999999729283, 11.05913360956146185, 18.21068369823747091 ) ) ;
#10365=CARTESIAN_POINT ( 'NONE',  ( 52.46643183416157541, 7.028187705514638672, 13.68930817193508531 ) ) ;
#10375=CARTESIAN_POINT ( 'NONE',  ( 55.53356816583845301, 11.31069182806492712, 17.97181229448534623 ) ) ;
#10384=CARTESIAN_POINT ( 'NONE',  ( 59.25000000000000711, 7.878679656440361612, 17.12132034355964549 ) ) ;
#10389=CARTESIAN_POINT ( 'NONE',  ( 58.12500000000000000, 12.12132034355964727, 17.12132034355963484 ) ) ;
#10398=CARTESIAN_POINT ( 'NONE',  ( 58.87500000000000711, 7.878679656440349177, 12.87867965644035984 ) ) ;
#10416=CARTESIAN_POINT ( 'NONE',  ( 56.18981816583843170, 9.931948859054346102, 10.99999999999999467 ) ) ;
#10433=CARTESIAN_POINT ( 'NONE',  ( 58.25231816583843170, 7.219692298483957771, 17.87654654797633924 ) ) ;
#10450=CARTESIAN_POINT ( 'NONE',  ( 57.18750000000000000, 9.999999999999989342, 11.99999999999999467 ) ) ;
#10462=CARTESIAN_POINT ( 'NONE',  ( 51.28125000000000000, 8.757359312880703683, 11.99999999999999822 ) ) ;
#10479=CARTESIAN_POINT ( 'NONE',  ( 59.31018183416157541, 14.00000000000000000, 15.06805114094561304 ) ) ;
#10490=CARTESIAN_POINT ( 'NONE',  ( 51.31481816583844591, 14.00000000000000178, 14.93194885905434610 ) ) ;
#10496=CARTESIAN_POINT ( 'NONE',  ( 57.28125000000000711, 8.757359312880703683, 11.99999999999999822 ) ) ;
#10499=CARTESIAN_POINT ( 'NONE',  ( 57.00000000000000000, 12.12132034355963484, 12.87867965644034740 ) ) ;
#10529=CARTESIAN_POINT ( 'NONE',  ( 51.75000000000000711, 7.171572875253819923, 17.82842712474619873 ) ) ;
#10540=VERTEX_POINT ( 'NONE', #5513 ) ;
#10549=CARTESIAN_POINT ( 'NONE',  ( 59.00231816583843170, 12.78030770151603868, 12.12345345202365188 ) ) ;
#10569=CARTESIAN_POINT ( 'NONE',  ( 56.25000000000000711, 7.878679656440361612, 17.12132034355964549 ) ) ;
#10592=CARTESIAN_POINT ( 'NONE',  ( 60.00000000000001421, 13.59380198783558669, 16.55161943776040800 ) ) ;
#10599=EDGE_LOOP ( 'NONE', ( #3231, #17560 ) ) ;
#10602=CARTESIAN_POINT ( 'NONE',  ( 59.21643183416158962, 13.97181229448536399, 16.72490539043799629 ) ) ;
#10613=CARTESIAN_POINT ( 'NONE',  ( 51.78356816583844591, 8.689308171935074654, 12.02818770551464489 ) ) ;
#10619=CARTESIAN_POINT ( 'NONE',  ( 56.43750000000000000, 10.00000000000000711, 17.99999999999999645 ) ) ;
#10621=CARTESIAN_POINT ( 'NONE',  ( 57.65625000000002132, 7.000000000000003553, 16.24264068711929099 ) ) ;
#10629=CARTESIAN_POINT ( 'NONE',  ( 57.93750000000000000, 10.00000000000000711, 17.99999999999999645 ) ) ;
#10647=CARTESIAN_POINT ( 'NONE',  ( 58.90856816583844591, 13.97181229448534978, 13.27509460956196641 ) ) ;
#10666=CARTESIAN_POINT ( 'NONE',  ( 52.78125000000000711, 8.343145750507600766, 11.00000000000000533 ) ) ;
#10675=CARTESIAN_POINT ( 'NONE',  ( 57.52893183416158962, 11.58880310854676132, 19.02818770551463956 ) ) ;
#10684=CARTESIAN_POINT ( 'NONE',  ( 58.40625000000000711, 12.99999999999999645, 13.75735931288070191 ) ) ;
#10686=DIRECTION ( 'NONE',  ( 0.000000000000000000, 0.000000000000000000, 1.000000000000000000 ) ) ;
#10701=CARTESIAN_POINT ( 'NONE',  ( 51.00000000000000711, 12.82842712474617741, 12.17157287525379239 ) ) ;
#10718=CARTESIAN_POINT ( 'NONE',  ( 56.77893183416158251, 8.411196891453236901, 10.97181229448535511 ) ) ;
#10730=CARTESIAN_POINT ( 'NONE',  ( 59.81250000000000711, 13.00000000000000000, 14.99999999999998757 ) ) ;
#10739=CARTESIAN_POINT ( 'NONE',  ( 56.06250000000000000, 6.999999999999997335, 15.00000000000000533 ) ) ;
#10744=CARTESIAN_POINT ( 'NONE',  ( 52.06481816583844591, 6.999999999999998224, 15.06805114094563436 ) ) ;
#10752=CARTESIAN_POINT ( 'NONE',  ( 53.81250000000000711, 13.00000000000000000, 14.99999999999998757 ) ) ;
#10770=CARTESIAN_POINT ( 'NONE',  ( 57.31481816583843170, 14.00000000000000178, 14.93194885905434610 ) ) ;
#10787=CARTESIAN_POINT ( 'NONE',  ( 54.75000000000000711, 7.171572875253819923, 17.82842712474619873 ) ) ;
#10796=CARTESIAN_POINT ( 'NONE',  ( 53.59143183416158962, 11.31069182806491291, 12.02818770551463778 ) ) ;
#10804=CARTESIAN_POINT ( 'NONE',  ( 59.62500000000000711, 12.12132034355964727, 17.12132034355963484 ) ) ;
#10834=CARTESIAN_POINT ( 'NONE',  ( 53.12268183416157541, 12.78030770151606177, 17.87654654797631792 ) ) ;
#10843=CARTESIAN_POINT ( 'NONE',  ( 52.06481816583844591, 6.999999999999998224, 15.06805114094563436 ) ) ;
#10848=CARTESIAN_POINT ( 'NONE',  ( 53.90625000000000000, 12.99999999999999645, 13.75735931288070191 ) ) ;
#10850=CARTESIAN_POINT ( 'NONE',  ( 53.43750000000000711, 10.00000000000000711, 17.99999999999999645 ) ) ;
#10858=CARTESIAN_POINT ( 'NONE',  ( 52.50000000000000711, 12.12132034355963484, 12.87867965644034740 ) ) ;
#10877=CARTESIAN_POINT ( 'NONE',  ( 51.46875000000000000, 5.999999999999987566, 13.34314575050763452 ) ) ;
#10891=CARTESIAN_POINT ( 'NONE',  ( 56.53125000000000711, 11.65685424949239923, 18.99999999999998934 ) ) ;
#10896=CARTESIAN_POINT ( 'NONE',  ( 51.28125000000000000, 8.343145750507600766, 11.00000000000000533 ) ) ;
#10905=CARTESIAN_POINT ( 'NONE',  ( 60.34143183416158962, 8.275094609562001935, 18.97181229448536044 ) ) ;
#10912=CARTESIAN_POINT ( 'NONE',  ( 56.34375000000000711, 8.757359312880723223, 18.00000000000000711 ) ) ;
#10944=CARTESIAN_POINT ( 'NONE',  ( 56.31018183416157541, 14.00000000000000000, 15.06805114094561304 ) ) ;
#10953=CARTESIAN_POINT ( 'NONE',  ( 53.47106816583843880, 6.971812294485350670, 13.82541045382635403 ) ) ;
#10960=CARTESIAN_POINT ( 'NONE',  ( 52.12500000000000711, 12.12132034355964727, 17.12132034355963484 ) ) ;
#10962=CARTESIAN_POINT ( 'NONE',  ( 51.93750000000000711, 10.00000000000000711, 17.99999999999999645 ) ) ;
#10970=CARTESIAN_POINT ( 'NONE',  ( 54.56250000000000711, 6.999999999999997335, 15.00000000000000533 ) ) ;
#10987=CARTESIAN_POINT ( 'NONE',  ( 52.62731816583844591, 12.87654654797634102, 17.78030770151602979 ) ) ;
#11002=CARTESIAN_POINT ( 'NONE',  ( 54.28125000000000000, 8.343145750507600766, 11.00000000000000355 ) ) ;
#11004=DIRECTION ( 'NONE',  ( 0.000000000000000000, -0.7071067811865406894, 0.7071067811865545671 ) ) ;
#11007=CARTESIAN_POINT ( 'NONE',  ( 53.75231816583844591, 7.219692298483957771, 17.87654654797633924 ) ) ;
#11009=CARTESIAN_POINT ( 'NONE',  ( 60.00000000000000711, 12.82842712474617741, 12.17157287525379239 ) ) ;
#11017=CARTESIAN_POINT ( 'NONE',  ( 56.21643183416158251, 13.97181229448536399, 16.72490539043799629 ) ) ;
#11027=CARTESIAN_POINT ( 'NONE',  ( 51.84375000000001421, 8.757359312880723223, 18.00000000000000711 ) ) ;
#11061=CARTESIAN_POINT ( 'NONE',  ( 56.12268183416157541, 12.78030770151606177, 17.87654654797631792 ) ) ;
#11070=CARTESIAN_POINT ( 'NONE',  ( 52.90856816583843880, 12.97181229448534978, 13.68930817193506755 ) ) ;
#11076=CARTESIAN_POINT ( 'NONE',  ( 52.21875000000002842, 13.00000000000000711, 16.24264068711927322 ) ) ;
#11079=CARTESIAN_POINT ( 'NONE',  ( 55.68750000000000000, 9.999999999999989342, 11.99999999999999467 ) ) ;
#11088=CARTESIAN_POINT ( 'NONE',  ( 55.40625000000000000, 12.99999999999999645, 13.75735931288070191 ) ) ;
#11095=COLOUR_RGB ( '', 0.31764706, 0.68627451, 0.89019608) ;
#11110=CARTESIAN_POINT ( 'NONE',  ( 54.50231816583843170, 12.78030770151603868, 12.12345345202365188 ) ) ;
#11127=CARTESIAN_POINT ( 'NONE',  ( 54.65625000000000711, 6.000000000000004441, 16.65685424949239390 ) ) ;
#11132=CARTESIAN_POINT ( 'NONE',  ( 54.68981816583844591, 9.931948859054346102, 10.99999999999999467 ) ) ;
#11142=CARTESIAN_POINT ( 'NONE',  ( 54.24768183416157541, 7.123453452023678523, 17.78030770151605822 ) ) ;
#11186=CARTESIAN_POINT ( 'NONE',  ( 54.81018183416157541, 14.00000000000000000, 15.06805114094561304 ) ) ;
#11194=CARTESIAN_POINT ( 'NONE',  ( 54.75000000000000711, 7.878679656440361612, 17.12132034355964549 ) ) ;
#11200=CARTESIAN_POINT ( 'NONE',  ( 51.09375000000000000, 11.24264068711927322, 11.99999999999998934 ) ) ;
#11202=CARTESIAN_POINT ( 'NONE',  ( 51.00000000000000711, 12.12132034355963484, 12.87867965644034740 ) ) ;
#11209=CARTESIAN_POINT ( 'NONE',  ( 51.28125000000000000, 8.757359312880703683, 11.99999999999999822 ) ) ;
#11225=CARTESIAN_POINT ( 'NONE',  ( 50.00231816583843170, 12.78030770151603868, 12.12345345202365188 ) ) ;
#11238=CARTESIAN_POINT ( 'NONE',  ( 55.40625000000000711, 13.99999999999999289, 13.34314575050759544 ) ) ;
#11243=CARTESIAN_POINT ( 'NONE',  ( 56.65856816583844591, 6.028187705514649330, 16.72490539043803182 ) ) ;
#11254=CARTESIAN_POINT ( 'NONE',  ( 55.93518183416157541, 9.931948859054379852, 18.99999999999999289 ) ) ;
#11301=CARTESIAN_POINT ( 'NONE',  ( 51.99768183416157541, 12.87654654797631792, 12.21969229848393113 ) ) ;
#11309=CARTESIAN_POINT ( 'NONE',  ( 55.96875000000000000, 6.999999999999992895, 13.75735931288071967 ) ) ;
#11319=CARTESIAN_POINT ( 'NONE',  ( 54.09375000000000711, 11.24264068711927322, 11.99999999999998934 ) ) ;
#11323=CARTESIAN_POINT ( 'NONE',  ( 55.87500000000000711, 7.878679656440349177, 12.87867965644035984 ) ) ;
#11332=CARTESIAN_POINT ( 'NONE',  ( 56.77893183416158251, 8.825410453826341595, 11.97181229448535511 ) ) ;
#11335=AXIS2_PLACEMENT_3D ( 'NONE', #6207, #454, #18783 ) ;
#11349=CARTESIAN_POINT ( 'NONE',  ( 58.34606816583844591, 8.825410453826357582, 18.02818770551464667 ) ) ;
#11362=CARTESIAN_POINT ( 'NONE',  ( 58.68750000000000000, 9.999999999999978684, 10.99999999999999645 ) ) ;
#11366=CARTESIAN_POINT ( 'NONE',  ( 54.50231816583843170, 12.78030770151603868, 12.12345345202365188 ) ) ;
#11373=CARTESIAN_POINT ( 'NONE',  ( 52.46643183416157541, 6.028187705514633343, 13.27509460956200016 ) ) ;
#11380=CARTESIAN_POINT ( 'NONE',  ( 51.00000000000000711, 12.12132034355963484, 12.87867965644034740 ) ) ;
#11422=CARTESIAN_POINT ( 'NONE',  ( 56.43750000000000000, 10.00000000000001776, 18.99999999999999645 ) ) ;
#11434=CARTESIAN_POINT ( 'NONE',  ( 58.03125000000000711, 11.24264068711929276, 18.00000000000000355 ) ) ;
#11441=CARTESIAN_POINT ( 'NONE',  ( 56.77893183416158251, 8.825410453826341595, 11.97181229448535511 ) ) ;
#11452=CARTESIAN_POINT ( 'NONE',  ( 57.90393183416158251, 13.02818770551463778, 13.82541045382633982 ) ) ;
#11474=CARTESIAN_POINT ( 'NONE',  ( 54.78356816583844591, 8.275094609561968184, 11.02818770551464667 ) ) ;
#11477=( NAMED_UNIT ( * ) SI_UNIT ( $, .STERADIAN. ) SOLID_ANGLE_UNIT ( ) );
#11497=CARTESIAN_POINT ( 'NONE',  ( 53.65856816583844591, 6.028187705514649330, 16.72490539043803182 ) ) ;
#11507=CARTESIAN_POINT ( 'NONE',  ( 55.56018183416157541, 5.999999999999996447, 14.93194885905437808 ) ) ;
#11549=CARTESIAN_POINT ( 'NONE',  ( 60.00000000000000711, 12.82842712474617741, 12.17157287525379239 ) ) ;
#11557=CARTESIAN_POINT ( 'NONE',  ( 54.93750000000000711, 10.00000000000000711, 17.99999999999999645 ) ) ;
#11562=CARTESIAN_POINT ( 'NONE',  ( 54.52893183416158962, 11.17458954617365663, 18.02818770551464311 ) ) ;
#11574=CARTESIAN_POINT ( 'NONE',  ( 60.34143183416158962, 8.689308171935088865, 17.97181229448535689 ) ) ;
#11591=CARTESIAN_POINT ( 'NONE',  ( 56.09606816583844591, 11.17458954617364242, 11.97181229448534800 ) ) ;
#11608=CARTESIAN_POINT ( 'NONE',  ( 52.31250000000000711, 14.00000000000000000, 14.99999999999997691 ) ) ;
#11616=CARTESIAN_POINT ( 'NONE',  ( 54.00000000000000711, 12.82842712474617741, 12.17157287525379239 ) ) ;
#11664=CARTESIAN_POINT ( 'NONE',  ( 58.50000000000000000, 12.82842712474617741, 12.17157287525379239 ) ) ;
#11671=CARTESIAN_POINT ( 'NONE',  ( 56.34375000000000711, 8.757359312880723223, 18.00000000000000355 ) ) ;
#11677=CARTESIAN_POINT ( 'NONE',  ( 59.59143183416158962, 11.31069182806491291, 12.02818770551463778 ) ) ;
#11686=CARTESIAN_POINT ( 'NONE',  ( 58.27893183416158962, 8.825410453826341595, 11.97181229448535511 ) ) ;
#11690=ORIENTED_EDGE ( 'NONE', *, *, #9539, .T. ) ;
#11706=CARTESIAN_POINT ( 'NONE',  ( 53.09606816583843170, 11.17458954617364242, 11.97181229448534800 ) ) ;
#11721=CARTESIAN_POINT ( 'NONE',  ( 52.87500000000000711, 7.171572875253794166, 12.17157287525381726 ) ) ;
#11735=CARTESIAN_POINT ( 'NONE',  ( 57.18750000000000000, 9.999999999999978684, 10.99999999999999645 ) ) ;
#11785=CARTESIAN_POINT ( 'NONE',  ( 52.21875000000002842, 13.00000000000000711, 16.24264068711927322 ) ) ;
#11794=CARTESIAN_POINT ( 'NONE',  ( 56.21643183416158251, 12.97181229448535689, 16.31069182806490758 ) ) ;
#11806=CARTESIAN_POINT ( 'NONE',  ( 59.96643183416158251, 7.028187705514638672, 13.68930817193508531 ) ) ;
#11823=CARTESIAN_POINT ( 'NONE',  ( 55.34606816583843880, 8.825410453826357582, 18.02818770551464667 ) ) ;
#11851=CARTESIAN_POINT ( 'NONE',  ( 56.90625000000000711, 13.99999999999999289, 13.34314575050759544 ) ) ;
#11875=AXIS2_PLACEMENT_3D ( 'NONE', #18753, #7985, #425 ) ;
#11917=CARTESIAN_POINT ( 'NONE',  ( 58.65393183416157541, 5.971812294485358663, 16.58880310854675599 ) ) ;
#11927=CARTESIAN_POINT ( 'NONE',  ( 52.27893183416158251, 8.825410453826341595, 11.97181229448535511 ) ) ;
#11940=CARTESIAN_POINT ( 'NONE',  ( 50.84606816583843880, 8.411196891453267099, 19.02818770551464667 ) ) ;
#11949=CARTESIAN_POINT ( 'NONE',  ( 52.34606816583843880, 8.825410453826357582, 18.02818770551464667 ) ) ;
#11971=CARTESIAN_POINT ( 'NONE',  ( 56.53125000000000711, 11.65685424949239923, 18.99999999999998934 ) ) ;
#12018=CARTESIAN_POINT ( 'NONE',  ( 52.40625000000000000, 12.99999999999999645, 13.75735931288070191 ) ) ;
#12028=CARTESIAN_POINT ( 'NONE',  ( 60.71643183416158962, 13.97181229448536399, 16.72490539043799629 ) ) ;
#12039=CARTESIAN_POINT ( 'NONE',  ( 58.46643183416158251, 6.028187705514633343, 13.27509460956200016 ) ) ;
#12047=CARTESIAN_POINT ( 'NONE',  ( 56.84606816583843880, 8.825410453826357582, 18.02818770551464667 ) ) ;
#12055=CARTESIAN_POINT ( 'NONE',  ( 57.93750000000000000, 10.00000000000000711, 17.99999999999999645 ) ) ;
#12059=CARTESIAN_POINT ( 'NONE',  ( 57.50231816583843170, 12.07320092032949610, 12.83056023321021044 ) ) ;
#12070=FILL_AREA_STYLE_COLOUR ( '', #11095 ) ;
#12086=CARTESIAN_POINT ( 'NONE',  ( 53.06250000000000711, 5.999999999999996447, 15.00000000000001599 ) ) ;
#12139=CARTESIAN_POINT ( 'NONE',  ( 60.00000000000003553, 13.52471821456362910, 16.68728994856221348 ) ) ;
#12150=CARTESIAN_POINT ( 'NONE',  ( 60.06018183416157541, 5.999999999999996447, 14.93194885905437808 ) ) ;
#12160=CARTESIAN_POINT ( 'NONE',  ( 56.37731816583843170, 7.830560233210212218, 12.92679907967049679 ) ) ;
#12167=CARTESIAN_POINT ( 'NONE',  ( 56.62500000000000000, 12.12132034355964727, 17.12132034355963484 ) ) ;
#12172=CARTESIAN_POINT ( 'NONE',  ( 59.90625000000000711, 12.99999999999999645, 13.75735931288070191 ) ) ;
#12182=CARTESIAN_POINT ( 'NONE',  ( 58.96875000000000711, 6.999999999999992895, 13.75735931288071967 ) ) ;
#12203=CARTESIAN_POINT ( 'NONE',  ( 57.87731816583843170, 7.123453452023657206, 12.21969229848395599 ) ) ;
#12225=CARTESIAN_POINT ( 'NONE',  ( 58.90856816583844591, 13.97181229448534978, 13.27509460956196641 ) ) ;
#12244=CARTESIAN_POINT ( 'NONE',  ( 60.00000000000000711, 12.12132034355963484, 12.87867965644034740 ) ) ;
#12257=CARTESIAN_POINT ( 'NONE',  ( 52.59375000000000711, 11.24264068711927322, 11.99999999999998934 ) ) ;
#12266=CARTESIAN_POINT ( 'NONE',  ( 60.00000000000004974, 13.73105986157044001, 13.57812919445311550 ) ) ;
#12276=CARTESIAN_POINT ( 'NONE',  ( 52.74768183416157541, 7.830560233210222876, 17.07320092032950498 ) ) ;
#12287=CARTESIAN_POINT ( 'NONE',  ( 55.81481816583843170, 12.99999999999999822, 14.93194885905435676 ) ) ;
#12295=CARTESIAN_POINT ( 'NONE',  ( 59.71875000000000711, 13.00000000000000711, 16.24264068711927322 ) ) ;
#12298=CARTESIAN_POINT ( 'NONE',  ( 58.87500000000000711, 7.878679656440349177, 12.87867965644035984 ) ) ;
#12324=CARTESIAN_POINT ( 'NONE',  ( 57.40856816583844591, 13.97181229448534978, 13.27509460956196641 ) ) ;
#12343=CARTESIAN_POINT ( 'NONE',  ( 57.87731816583843170, 7.123453452023657206, 12.21969229848395599 ) ) ;
#12360=CARTESIAN_POINT ( 'NONE',  ( 57.84375000000000711, 8.757359312880723223, 18.00000000000000711 ) ) ;
#12380=CARTESIAN_POINT ( 'NONE',  ( 60.00000000000004974, 12.97738825490581682, 15.73700537498047503 ) ) ;
#12389=CARTESIAN_POINT ( 'NONE',  ( 59.87268183416157541, 7.219692298483935566, 12.12345345202367675 ) ) ;
#12400=CARTESIAN_POINT ( 'NONE',  ( 58.81481816583843170, 12.99999999999999822, 14.93194885905435676 ) ) ;
#12406=CARTESIAN_POINT ( 'NONE',  ( 59.90625000000000711, 12.99999999999999645, 13.75735931288070191 ) ) ;
#12408=CARTESIAN_POINT ( 'NONE',  ( 50.56481816583844591, 6.999999999999998224, 15.06805114094563436 ) ) ;
#12436=CARTESIAN_POINT ( 'NONE',  ( 52.87500000000000711, 7.171572875253794166, 12.17157287525381726 ) ) ;
#12457=CARTESIAN_POINT ( 'NONE',  ( 55.03125000000000000, 11.65685424949239923, 18.99999999999998934 ) ) ;
#12469=CARTESIAN_POINT ( 'NONE',  ( 58.93518183416157541, 9.931948859054379852, 18.99999999999999289 ) ) ;
#12478=CARTESIAN_POINT ( 'NONE',  ( 58.31250000000000000, 13.00000000000000000, 14.99999999999998757 ) ) ;
#12505=CARTESIAN_POINT ( 'NONE',  ( 60.00000000000002842, 13.86373736226824427, 15.83363142472004448 ) ) ;
#12514=CARTESIAN_POINT ( 'NONE',  ( 55.18518183416157541, 10.06805114094561659, 10.99999999999999645 ) ) ;
#12524=CARTESIAN_POINT ( 'NONE',  ( 50.18981816583844591, 9.931948859054354983, 11.99999999999999645 ) ) ;
#12531=CARTESIAN_POINT ( 'NONE',  ( 58.40625000000000711, 12.99999999999999645, 13.75735931288070191 ) ) ;
#12533=CARTESIAN_POINT ( 'NONE',  ( 57.56250000000000000, 6.999999999999997335, 15.00000000000000533 ) ) ;
#12542=CARTESIAN_POINT ( 'NONE',  ( 57.28125000000000711, 8.757359312880703683, 11.99999999999999822 ) ) ;
#12563=CARTESIAN_POINT ( 'NONE',  ( 51.28125000000000000, 8.343145750507600766, 11.00000000000000533 ) ) ;
#12565=SURFACE_STYLE_FILL_AREA ( #5220 ) ;
#12582=CARTESIAN_POINT ( 'NONE',  ( 51.84375000000001421, 8.343145750507638070, 19.00000000000000711 ) ) ;
#12591=ADVANCED_FACE ( 'NONE', ( #21120 ), #19777, .T. ) ;
#12595=CARTESIAN_POINT ( 'NONE',  ( 58.18518183416157541, 10.06805114094561659, 10.99999999999999645 ) ) ;
#12602=CARTESIAN_POINT ( 'NONE',  ( 54.93750000000000711, 10.00000000000000711, 17.99999999999999645 ) ) ;
#12625=CARTESIAN_POINT ( 'NONE',  ( 60.00000000000004974, 12.13806810308082440, 17.37563432761511706 ) ) ;
#12638=CARTESIAN_POINT ( 'NONE',  ( 56.68518183416157541, 10.06805114094561659, 10.99999999999999645 ) ) ;
#12647=CARTESIAN_POINT ( 'NONE',  ( 50.28356816583843880, 8.689308171935074654, 12.02818770551464489 ) ) ;
#12652=CARTESIAN_POINT ( 'NONE',  ( 60.81018183416157541, 12.99999999999999822, 15.06805114094562192 ) ) ;
#12656=CARTESIAN_POINT ( 'NONE',  ( 53.06250000000000711, 6.999999999999997335, 15.00000000000000533 ) ) ;
#12667=CARTESIAN_POINT ( 'NONE',  ( 55.12500000000000711, 12.12132034355964727, 17.12132034355963484 ) ) ;
#12688=CARTESIAN_POINT ( 'NONE',  ( 55.90856816583843880, 13.97181229448534978, 13.27509460956196641 ) ) ;
#12702=CARTESIAN_POINT ( 'NONE',  ( 56.90625000000000711, 13.99999999999999289, 13.34314575050759544 ) ) ;
#12707=CARTESIAN_POINT ( 'NONE',  ( 51.46875000000000000, 5.999999999999987566, 13.34314575050763452 ) ) ;
#12715=CARTESIAN_POINT ( 'NONE',  ( 60.99768183416157541, 12.87654654797631792, 12.21969229848393113 ) ) ;
#12722=CARTESIAN_POINT ( 'NONE',  ( 58.87500000000000711, 7.878679656440349177, 12.87867965644035984 ) ) ;
#12751=CARTESIAN_POINT ( 'NONE',  ( 54.34143183416158251, 8.275094609562001935, 18.97181229448536044 ) ) ;
#12759=CARTESIAN_POINT ( 'NONE',  ( 53.93981816583844591, 10.06805114094563791, 17.99999999999999645 ) ) ;
#12766=CARTESIAN_POINT ( 'NONE',  ( 60.43518183416157541, 9.931948859054372747, 17.99999999999999645 ) ) ;
#12768=CARTESIAN_POINT ( 'NONE',  ( 54.37500000000000711, 7.878679656440349177, 12.87867965644035984 ) ) ;
#12776=CARTESIAN_POINT ( 'NONE',  ( 54.28125000000000000, 8.757359312880703683, 11.99999999999999822 ) ) ;
#12795=CARTESIAN_POINT ( 'NONE',  ( 53.00231816583844591, 12.78030770151603868, 12.12345345202365188 ) ) ;
#12806=ORIENTED_EDGE ( 'NONE', *, *, #7596, .F. ) ;
#12807=CARTESIAN_POINT ( 'NONE',  ( 54.09375000000000711, 11.65685424949236015, 10.99999999999998579 ) ) ;
#12811=CARTESIAN_POINT ( 'NONE',  ( 52.43981816583844591, 10.06805114094564857, 19.00000000000000000 ) ) ;
#12814=LINE ( 'NONE', #11009, #22921 ) ;
#12821=CARTESIAN_POINT ( 'NONE',  ( 53.31018183416157541, 14.00000000000000000, 15.06805114094561304 ) ) ;
#12828=CARTESIAN_POINT ( 'NONE',  ( 52.87500000000000711, 7.878679656440349177, 12.87867965644035984 ) ) ;
#12860=CARTESIAN_POINT ( 'NONE',  ( 57.34143183416159673, 8.275094609562001935, 18.97181229448536044 ) ) ;
#12870=CARTESIAN_POINT ( 'NONE',  ( 51.22106816583844591, 13.02818770551464489, 16.17458954617363531 ) ) ;
#12875=CARTESIAN_POINT ( 'NONE',  ( 51.75000000000000711, 7.878679656440361612, 17.12132034355964549 ) ) ;
#12878=CARTESIAN_POINT ( 'NONE',  ( 54.00000000000000711, 12.12132034355963484, 12.87867965644034740 ) ) ;
#12886=CARTESIAN_POINT ( 'NONE',  ( 52.12500000000000711, 12.12132034355964727, 17.12132034355963484 ) ) ;
#12902=CARTESIAN_POINT ( 'NONE',  ( 50.18981816583844591, 9.931948859054346102, 10.99999999999999467 ) ) ;
#12918=CARTESIAN_POINT ( 'NONE',  ( 57.75000000000000000, 7.171572875253819923, 17.82842712474619873 ) ) ;
#12924=CARTESIAN_POINT ( 'NONE',  ( 51.59606816583843170, 11.58880310854672935, 10.97181229448534445 ) ) ;
#12933=CARTESIAN_POINT ( 'NONE',  ( 56.59143183416158962, 11.72490539043799984, 11.02818770551463246 ) ) ;
#12942=CARTESIAN_POINT ( 'NONE',  ( 52.21875000000001421, 13.00000000000000533, 16.24264068711927322 ) ) ;
#12980=CARTESIAN_POINT ( 'NONE',  ( 57.06018183416157541, 5.999999999999996447, 14.93194885905437808 ) ) ;
#12988=CARTESIAN_POINT ( 'NONE',  ( 54.28125000000000000, 8.757359312880703683, 11.99999999999999822 ) ) ;
#12996=CARTESIAN_POINT ( 'NONE',  ( 51.00000000000000711, 12.12132034355963484, 12.87867965644034740 ) ) ;
#12997=CARTESIAN_POINT ( 'NONE',  ( 52.68750000000000711, 9.999999999999989342, 11.99999999999999467 ) ) ;
#13006=CARTESIAN_POINT ( 'NONE',  ( 51.37500000000000711, 7.878679656440349177, 12.87867965644035984 ) ) ;
#13028=CARTESIAN_POINT ( 'NONE',  ( 53.84606816583843880, 8.411196891453267099, 19.02818770551464667 ) ) ;
#13042=CARTESIAN_POINT ( 'NONE',  ( 55.12500000000000711, 12.82842712474620228, 17.82842712474617386 ) ) ;
#13047=CARTESIAN_POINT ( 'NONE',  ( 54.31481816583844591, 14.00000000000000178, 14.93194885905434610 ) ) ;
#13059=CARTESIAN_POINT ( 'NONE',  ( 56.02893183416158962, 11.58880310854676132, 19.02818770551463956 ) ) ;
#13067=CARTESIAN_POINT ( 'NONE',  ( 53.62500000000000711, 12.12132034355964727, 17.12132034355963484 ) ) ;
#13101=CARTESIAN_POINT ( 'NONE',  ( 57.46875000000000711, 5.999999999999987566, 13.34314575050763452 ) ) ;
#13109=CARTESIAN_POINT ( 'NONE',  ( 53.71875000000002132, 13.00000000000000711, 16.24264068711927322 ) ) ;
#13116=CARTESIAN_POINT ( 'NONE',  ( 54.00000000000000711, 12.12132034355963484, 12.87867965644034740 ) ) ;
#13118=CARTESIAN_POINT ( 'NONE',  ( 54.56250000000000711, 6.999999999999997335, 15.00000000000000533 ) ) ;
#13126=CARTESIAN_POINT ( 'NONE',  ( 54.75000000000000711, 7.878679656440361612, 17.12132034355964549 ) ) ;
#13140=CARTESIAN_POINT ( 'NONE',  ( 58.53356816583845301, 11.31069182806492712, 17.97181229448534623 ) ) ;
#13155=CARTESIAN_POINT ( 'NONE',  ( 55.96875000000001421, 5.999999999999987566, 13.34314575050763452 ) ) ;
#13160=CARTESIAN_POINT ( 'NONE',  ( 52.25231816583844591, 7.219692298483957771, 17.87654654797633924 ) ) ;
#13168=CARTESIAN_POINT ( 'NONE',  ( 52.84143183416158251, 8.275094609562001935, 18.97181229448536044 ) ) ;
#13178=CARTESIAN_POINT ( 'NONE',  ( 52.03125000000000711, 11.24264068711929276, 18.00000000000000000 ) ) ;
#13213=CARTESIAN_POINT ( 'NONE',  ( 56.81250000000000000, 14.00000000000000000, 14.99999999999997691 ) ) ;
#13223=CARTESIAN_POINT ( 'NONE',  ( 55.31250000000000711, 13.00000000000000000, 14.99999999999998757 ) ) ;
#13231=CARTESIAN_POINT ( 'NONE',  ( 59.40393183416158251, 13.02818770551463778, 13.82541045382633982 ) ) ;
#13233=( BOUNDED_CURVE ( )  B_SPLINE_CURVE ( 2, ( #19837, #19489, #3087, #6805, #5010, #3198, #17821, #1387, #8727, #23323, #1982, #8982, #3554, #20302, #11362, #192, #16270, #9321, #4027, #18405, #3787, #18637, #20064, #16383, #12918, #16613, #23562, #14485, #7522, #2099, #20417, #7168, #7296, #12702, #21747, #5359, #14837, #10891, #5592, #22093, #9215, #19955, #18170, #13155, #1753, #9089, #14605, #5710, #3904, #11238, #23680, #21977, #13042, #5828, #7409, #18513, #9437, #11127, #5471, #16729, #312, #11002, #21866, #12807, #3667, #1867, #18284, #16500, #7646, #14964, #75, #14719, #20181, #22217, #10046, #9795, #11721, #18989, #2224, #20541, #13628, #21011, #11608, #22699, #4271, #2575, #17334, #6429, #4628, #13400, #9680, #6194, #9921, #9565, #7760, #17217, #19116 ),
 .UNSPECIFIED., .F., .F. ) 
 B_SPLINE_CURVE_WITH_KNOTS ( ( 3, 2, 2, 2, 2, 2, 2, 2, 2, 2, 2, 2, 2, 2, 2, 2, 2, 2, 2, 2, 2, 2, 2, 2, 2, 2, 2, 2, 2, 2, 2, 2, 2, 2, 2, 2, 2, 2, 2, 2, 2, 2, 2, 2, 2, 2, 2, 2, 3 ),
 ( 0.000000000000000000, 0.02083333333333333218, 0.04166666666666666435, 0.06250000000000000000, 0.08333333333333332871, 0.1041666666666666713, 0.1250000000000000000, 0.1458333333333333426, 0.1666666666666666574, 0.1875000000000000000, 0.2083333333333333426, 0.2291666666666666574, 0.2500000000000000000, 0.2708333333333333148, 0.2916666666666666852, 0.3125000000000000000, 0.3333333333333333148, 0.3541666666666666852, 0.3750000000000000000, 0.3958333333333333148, 0.4166666666666666852, 0.4375000000000000000, 0.4583333333333333148, 0.4791666666666666852, 0.5000000000000000000, 0.5208333333333333703, 0.5416666666666666297, 0.5625000000000000000, 0.5833333333333333703, 0.6041666666666666297, 0.6250000000000000000, 0.6458333333333333703, 0.6666666666666666297, 0.6875000000000000000, 0.7083333333333333703, 0.7291666666666666297, 0.7500000000000000000, 0.7708333333333333703, 0.7916666666666666297, 0.8125000000000000000, 0.8333333333333333703, 0.8541666666666666297, 0.8750000000000000000, 0.8958333333333333703, 0.9166666666666666297, 0.9375000000000000000, 0.9583333333333333703, 0.9791666666666666297, 1.000000000000000000 ),
 .UNSPECIFIED. ) 
 CURVE ( )  GEOMETRIC_REPRESENTATION_ITEM ( )  RATIONAL_B_SPLINE_CURVE ( ( 1.000000000000000000, 0.9238795325112867385, 1.000000000000000000, 0.9238795325112867385, 1.000000000000000000, 0.9238795325112867385, 1.000000000000000000, 0.9238795325112867385, 1.000000000000000000, 0.9238795325112867385, 1.000000000000000000, 0.9238795325112867385, 1.000000000000000000, 0.9238795325112867385, 1.000000000000000000, 0.9238795325112867385, 1.000000000000000000, 0.9238795325112867385, 1.000000000000000000, 0.9238795325112867385, 1.000000000000000000, 0.9238795325112867385, 1.000000000000000000, 0.9238795325112867385, 1.000000000000000000, 0.9238795325112867385, 1.000000000000000000, 0.9238795325112867385, 1.000000000000000000, 0.9238795325112867385, 1.000000000000000000, 0.9238795325112867385, 1.000000000000000000, 0.9238795325112867385, 1.000000000000000000, 0.9238795325112867385, 1.000000000000000000, 0.9238795325112867385, 1.000000000000000000, 0.9238795325112867385, 1.000000000000000000, 0.9238795325112867385, 1.000000000000000000, 0.9238795325112867385, 1.000000000000000000, 0.9238795325112867385, 1.000000000000000000, 0.9238795325112867385, 1.000000000000000000, 0.9238795325112867385, 1.000000000000000000, 0.9238795325112867385, 1.000000000000000000, 0.9238795325112867385, 1.000000000000000000, 0.9238795325112867385, 1.000000000000000000, 0.9238795325112867385, 1.000000000000000000, 0.9238795325112867385, 1.000000000000000000, 0.9238795325112867385, 1.000000000000000000, 0.9238795325112867385, 1.000000000000000000, 0.9238795325112867385, 1.000000000000000000, 0.9238795325112867385, 1.000000000000000000, 0.9238795325112867385, 1.000000000000000000, 0.9238795325112867385, 1.000000000000000000, 0.9238795325112867385, 1.000000000000000000, 0.9238795325112867385, 1.000000000000000000, 0.9238795325112867385, 1.000000000000000000, 0.9238795325112867385, 1.000000000000000000, 0.9238795325112867385, 1.000000000000000000, 0.9238795325112867385, 1.000000000000000000, 0.9238795325112867385, 1.000000000000000000, 0.9238795325112867385, 1.000000000000000000, 0.9238795325112867385, 1.000000000000000000, 0.9238795325112867385, 1.000000000000000000, 0.9238795325112867385, 1.000000000000000000, 0.9238795325112867385, 1.000000000000000000 ) ) 
 REPRESENTATION_ITEM ( '' )  );
#13241=CARTESIAN_POINT ( 'NONE',  ( 59.49768183416157541, 12.16943976678977535, 12.92679907967048614 ) ) ;
#13261=CARTESIAN_POINT ( 'NONE',  ( 50.37731816583844591, 7.123453452023657206, 12.21969229848395599 ) ) ;
#13278=CARTESIAN_POINT ( 'NONE',  ( 53.28356816583845301, 8.275094609561968184, 11.02818770551464667 ) ) ;
#13288=CARTESIAN_POINT ( 'NONE',  ( 52.74768183416157541, 7.123453452023678523, 17.78030770151605822 ) ) ;
#13294=CARTESIAN_POINT ( 'NONE',  ( 53.71875000000000711, 13.00000000000000533, 16.24264068711927322 ) ) ;
#13332=CARTESIAN_POINT ( 'NONE',  ( 57.75000000000000000, 7.171572875253819923, 17.82842712474619873 ) ) ;
#13342=CARTESIAN_POINT ( 'NONE',  ( 57.46875000000000711, 6.999999999999992895, 13.75735931288071967 ) ) ;
#13350=CARTESIAN_POINT ( 'NONE',  ( 54.90393183416157541, 13.02818770551463778, 13.82541045382633982 ) ) ;
#13361=CARTESIAN_POINT ( 'NONE',  ( 56.12268183416157541, 12.07320092032950676, 17.16943976678977180 ) ) ;
#13369=CARTESIAN_POINT ( 'NONE',  ( 60.00000000000000711, 12.47487373415290612, 12.52512626584706901 ) ) ;
#13384=CARTESIAN_POINT ( 'NONE',  ( 55.15856816583844591, 7.028187705514647554, 16.31069182806492179 ) ) ;
#13389=CARTESIAN_POINT ( 'NONE',  ( 58.50000000000000000, 12.12132034355963484, 12.87867965644034740 ) ) ;
#13400=CARTESIAN_POINT ( 'NONE',  ( 51.65625000000000711, 6.000000000000004441, 16.65685424949239390 ) ) ;
#13411=CARTESIAN_POINT ( 'NONE',  ( 54.65625000000001421, 6.000000000000004441, 16.65685424949239390 ) ) ;
#13457=CARTESIAN_POINT ( 'NONE',  ( 55.68750000000000000, 9.999999999999978684, 10.99999999999999645 ) ) ;
#13459=PRODUCT_CONTEXT ( 'NONE', #1177, 'mechanical' ) ;
#13467=CARTESIAN_POINT ( 'NONE',  ( 56.25000000000000711, 7.878679656440361612, 17.12132034355964549 ) ) ;
#13472=CARTESIAN_POINT ( 'NONE',  ( 53.96643183416157541, 7.028187705514638672, 13.68930817193508531 ) ) ;
#13482=CARTESIAN_POINT ( 'NONE',  ( 59.68518183416157541, 10.06805114094562548, 11.99999999999999645 ) ) ;
#13500=CARTESIAN_POINT ( 'NONE',  ( 55.43981816583843170, 10.06805114094563791, 17.99999999999999645 ) ) ;
#13522=CARTESIAN_POINT ( 'NONE',  ( 55.12500000000000711, 12.82842712474620228, 17.82842712474617386 ) ) ;
#13581=CARTESIAN_POINT ( 'NONE',  ( 57.06018183416157541, 7.000000000000000000, 14.93194885905437097 ) ) ;
#13591=CARTESIAN_POINT ( 'NONE',  ( 51.00000000000000711, 12.12132034355963484, 12.87867965644034740 ) ) ;
#13612=CARTESIAN_POINT ( 'NONE',  ( 53.84606816583843880, 8.825410453826357582, 18.02818770551464667 ) ) ;
#13628=CARTESIAN_POINT ( 'NONE',  ( 52.50000000000000711, 12.82842712474617741, 12.17157287525379239 ) ) ;
#13638=CARTESIAN_POINT ( 'NONE',  ( 54.84375000000000000, 8.343145750507638070, 19.00000000000000711 ) ) ;
#13698=CARTESIAN_POINT ( 'NONE',  ( 58.84143183416158962, 8.689308171935088865, 17.97181229448535689 ) ) ;
#13710=CARTESIAN_POINT ( 'NONE',  ( 51.09375000000000000, 11.24264068711927322, 11.99999999999998934 ) ) ;
#13720=CARTESIAN_POINT ( 'NONE',  ( 54.87731816583843170, 7.830560233210212218, 12.92679907967049679 ) ) ;
#13731=CARTESIAN_POINT ( 'NONE',  ( 54.50231816583843170, 12.07320092032949610, 12.83056023321021044 ) ) ;
#13740=FILL_AREA_STYLE ('',( #12070 ) ) ;
#13756=PRODUCT ( 'End Stop Bumper spring', 'End Stop Bumper spring', '', ( #13459 ) ) ;
#13758=PRODUCT_DEFINITION_FORMATION_WITH_SPECIFIED_SOURCE ( 'ANY', '', #13756, .NOT_KNOWN. ) ;
#13762=CARTESIAN_POINT ( 'NONE',  ( 56.81250000000000000, 14.00000000000000000, 14.99999999999997691 ) ) ;
#13773=EDGE_LOOP ( 'NONE', ( #12806, #7927, #13971, #3023 ) ) ;
#13818=CARTESIAN_POINT ( 'NONE',  ( 51.56250000000000711, 6.999999999999997335, 15.00000000000000533 ) ) ;
#13826=CARTESIAN_POINT ( 'NONE',  ( 57.99768183416157541, 12.87654654797631792, 12.21969229848393113 ) ) ;
#13837=CARTESIAN_POINT ( 'NONE',  ( 59.02893183416158251, 11.58880310854676132, 19.02818770551463956 ) ) ;
#13846=CARTESIAN_POINT ( 'NONE',  ( 55.43981816583843170, 10.06805114094563791, 17.99999999999999645 ) ) ;
#13855=CARTESIAN_POINT ( 'NONE',  ( 57.40856816583844591, 12.97181229448534978, 13.68930817193506755 ) ) ;
#13870=CARTESIAN_POINT ( 'NONE',  ( 60.00000000000000711, 15.00000000000000000, 10.00000000000007105 ) ) ;
#13871=ORIENTED_EDGE ( 'NONE', *, *, #2088, .T. ) ;
#13879=CARTESIAN_POINT ( 'NONE',  ( 54.56250000000000711, 5.999999999999996447, 15.00000000000001599 ) ) ;
#13937=CARTESIAN_POINT ( 'NONE',  ( 60.00000000000000711, 11.02940789746247141, 18.43681100577745013 ) ) ;
#13948=CARTESIAN_POINT ( 'NONE',  ( 60.52893183416158251, 11.58880310854676132, 19.02818770551463956 ) ) ;
#13956=CARTESIAN_POINT ( 'NONE',  ( 57.40856816583844591, 12.97181229448534978, 13.68930817193506755 ) ) ;
#13962=CARTESIAN_POINT ( 'NONE',  ( 57.56250000000000000, 6.999999999999997335, 15.00000000000000533 ) ) ;
#13965=CARTESIAN_POINT ( 'NONE',  ( 57.75000000000000000, 7.878679656440361612, 17.12132034355964549 ) ) ;
#13971=ORIENTED_EDGE ( 'NONE', *, *, #4996, .T. ) ;
#13975=CARTESIAN_POINT ( 'NONE',  ( 59.34375000000000711, 8.757359312880723223, 18.00000000000000355 ) ) ;
#13989=CARTESIAN_POINT ( 'NONE',  ( 51.65625000000000711, 6.000000000000004441, 16.65685424949239390 ) ) ;
#14009=CARTESIAN_POINT ( 'NONE',  ( 53.90625000000000000, 13.99999999999999289, 13.34314575050759544 ) ) ;
#14042=CARTESIAN_POINT ( 'NONE',  ( 60.00000000000002842, 13.36943630122111415, 16.95040930672855595 ) ) ;
#14052=CARTESIAN_POINT ( 'NONE',  ( 53.21643183416158251, 12.97181229448535689, 16.31069182806490758 ) ) ;
#14066=CARTESIAN_POINT ( 'NONE',  ( 55.72106816583844591, 13.02818770551464489, 16.17458954617363531 ) ) ;
#14080=CARTESIAN_POINT ( 'NONE',  ( 50.47106816583844591, 6.971812294485350670, 13.82541045382635403 ) ) ;
#14088=CARTESIAN_POINT ( 'NONE',  ( 58.12500000000000000, 12.12132034355964727, 17.12132034355963484 ) ) ;
#14089=( NAMED_UNIT ( * ) SI_UNIT ( $, .STERADIAN. ) SOLID_ANGLE_UNIT ( ) );
#14111=CARTESIAN_POINT ( 'NONE',  ( 55.15856816583844591, 6.028187705514649330, 16.72490539043803182 ) ) ;
#14130=CARTESIAN_POINT ( 'NONE',  ( 53.81250000000000711, 14.00000000000000000, 14.99999999999997691 ) ) ;
#14147=CARTESIAN_POINT ( 'NONE',  ( 58.03125000000000711, 11.24264068711929276, 18.00000000000000000 ) ) ;
#14172=CARTESIAN_POINT ( 'NONE',  ( 60.00000000000000000, 11.54527125603259030, 17.88342085427740713 ) ) ;
#14183=CARTESIAN_POINT ( 'NONE',  ( 60.43518183416157541, 9.931948859054379852, 18.99999999999999289 ) ) ;
#14195=CARTESIAN_POINT ( 'NONE',  ( 58.43981816583843170, 10.06805114094563791, 17.99999999999999645 ) ) ;
#14201=CARTESIAN_POINT ( 'NONE',  ( 58.78125000000000711, 8.757359312880703683, 11.99999999999999822 ) ) ;
#14205=CARTESIAN_POINT ( 'NONE',  ( 59.81250000000000711, 13.00000000000000000, 14.99999999999998757 ) ) ;
#14214=CARTESIAN_POINT ( 'NONE',  ( 57.46875000000000711, 6.999999999999992895, 13.75735931288071967 ) ) ;
#14228=ORIENTED_EDGE ( 'NONE', *, *, #4996, .F. ) ;
#14234=CARTESIAN_POINT ( 'NONE',  ( 56.09606816583844591, 11.58880310854672935, 10.97181229448534445 ) ) ;
#14254=CARTESIAN_POINT ( 'NONE',  ( 53.06250000000000711, 5.999999999999996447, 15.00000000000001599 ) ) ;
#14261=CARTESIAN_POINT ( 'NONE',  ( 52.18518183416157541, 10.06805114094562548, 11.99999999999999645 ) ) ;
#14269=CARTESIAN_POINT ( 'NONE',  ( 57.28125000000000711, 8.757359312880703683, 11.99999999999999822 ) ) ;
#14290=CARTESIAN_POINT ( 'NONE',  ( 60.00000000000000000, 12.03166802832783766, 18.18714555911078889 ) ) ;
#14299=CARTESIAN_POINT ( 'NONE',  ( 55.65393183416158251, 5.971812294485358663, 16.58880310854675599 ) ) ;
#14310=CARTESIAN_POINT ( 'NONE',  ( 53.75231816583844591, 7.926799079670502124, 17.16943976678978245 ) ) ;
#14318=CARTESIAN_POINT ( 'NONE',  ( 55.87500000000000711, 7.878679656440349177, 12.87867965644035984 ) ) ;
#14320=CARTESIAN_POINT ( 'NONE',  ( 56.53125000000000711, 11.24264068711929276, 18.00000000000000355 ) ) ;
#14336=PLANE ( 'NONE',  #16770 ) ;
#14350=CARTESIAN_POINT ( 'NONE',  ( 52.21875000000002842, 14.00000000000000888, 16.65685424949235482 ) ) ;
#14369=CARTESIAN_POINT ( 'NONE',  ( 54.84375000000000000, 8.343145750507638070, 19.00000000000000711 ) ) ;
#14381=CARTESIAN_POINT ( 'NONE',  ( 57.24768183416158962, 7.123453452023678523, 17.78030770151605822 ) ) ;
#14387=CARTESIAN_POINT ( 'NONE',  ( 55.96875000000001421, 6.999999999999992006, 13.75735931288071967 ) ) ;
#14411=CARTESIAN_POINT ( 'NONE',  ( 59.99999999999995026, 12.29613458025714401, 18.03534775876610752 ) ) ;
#14421=CARTESIAN_POINT ( 'NONE',  ( 53.49768183416157541, 12.87654654797631792, 12.21969229848393113 ) ) ;
#14430=CARTESIAN_POINT ( 'NONE',  ( 59.25000000000000711, 7.878679656440361612, 17.12132034355964549 ) ) ;
#14435=CARTESIAN_POINT ( 'NONE',  ( 52.40625000000000000, 12.99999999999999645, 13.75735931288070191 ) ) ;
#14437=CARTESIAN_POINT ( 'NONE',  ( 59.25000000000000711, 7.878679656440361612, 17.12132034355964549 ) ) ;
#14447=CARTESIAN_POINT ( 'NONE',  ( 54.65625000000001421, 7.000000000000003553, 16.24264068711929099 ) ) ;
#14466=CARTESIAN_POINT ( 'NONE',  ( 57.03356816583845301, 11.72490539043803004, 18.97181229448534268 ) ) ;
#14468=SURFACE_SIDE_STYLE ('',( #12565 ) ) ;
#14485=CARTESIAN_POINT ( 'NONE',  ( 57.46875000000000711, 5.999999999999987566, 13.34314575050763452 ) ) ;
#14489=CARTESIAN_POINT ( 'NONE',  ( 52.03124999999999289, 11.65685424949239923, 18.99999999999998934 ) ) ;
#14500=CARTESIAN_POINT ( 'NONE',  ( 52.09143183416158251, 11.31069182806491291, 12.02818770551463778 ) ) ;
#14509=CARTESIAN_POINT ( 'NONE',  ( 54.28125000000000000, 8.757359312880703683, 11.99999999999999822 ) ) ;
#14546=CARTESIAN_POINT ( 'NONE',  ( 55.46643183416158962, 6.028187705514633343, 13.27509460956200016 ) ) ;
#14556=CARTESIAN_POINT ( 'NONE',  ( 53.00231816583844591, 12.07320092032949610, 12.83056023321021044 ) ) ;
#14562=CARTESIAN_POINT ( 'NONE',  ( 55.31250000000000711, 13.00000000000000000, 14.99999999999998757 ) ) ;
#14566=CARTESIAN_POINT ( 'NONE',  ( 53.90625000000000000, 12.99999999999999645, 13.75735931288070191 ) ) ;
#14573=CARTESIAN_POINT ( 'NONE',  ( 52.40625000000000000, 12.99999999999999645, 13.75735931288070191 ) ) ;
#14593=CARTESIAN_POINT ( 'NONE',  ( 53.56481816583844591, 5.999999999999996447, 15.06805114094564502 ) ) ;
#14605=CARTESIAN_POINT ( 'NONE',  ( 55.68750000000000000, 9.999999999999978684, 10.99999999999999645 ) ) ;
#14609=CARTESIAN_POINT ( 'NONE',  ( 55.62731816583843170, 12.87654654797634102, 17.78030770151602979 ) ) ;
#14618=CARTESIAN_POINT ( 'NONE',  ( 59.49768183416157541, 12.87654654797631792, 12.21969229848393113 ) ) ;
#14626=CARTESIAN_POINT ( 'NONE',  ( 55.40625000000000711, 12.99999999999999645, 13.75735931288070191 ) ) ;
#14659=CARTESIAN_POINT ( 'NONE',  ( 57.90393183416158251, 14.02818770551463956, 13.41119689145323335 ) ) ;
#14667=CARTESIAN_POINT ( 'NONE',  ( 51.59606816583843170, 11.17458954617364242, 11.97181229448534800 ) ) ;
#14675=CARTESIAN_POINT ( 'NONE',  ( 52.96875000000000000, 6.999999999999992895, 13.75735931288071967 ) ) ;
#14679=CARTESIAN_POINT ( 'NONE',  ( 55.40625000000000000, 12.99999999999999645, 13.75735931288070191 ) ) ;
#14687=CARTESIAN_POINT ( 'NONE',  ( 54.37500000000000711, 7.878679656440349177, 12.87867965644035984 ) ) ;
#14706=CARTESIAN_POINT ( 'NONE',  ( 52.15856816583843880, 6.028187705514649330, 16.72490539043803182 ) ) ;
#14719=CARTESIAN_POINT ( 'NONE',  ( 53.34375000000000000, 8.343145750507636293, 19.00000000000000000 ) ) ;
#14723=CARTESIAN_POINT ( 'NONE',  ( 53.09606816583843170, 11.58880310854672935, 10.97181229448534445 ) ) ;
#14733=CARTESIAN_POINT ( 'NONE',  ( 59.25000000000000711, 7.171572875253819923, 17.82842712474619873 ) ) ;
#14777=CARTESIAN_POINT ( 'NONE',  ( 57.24768183416158962, 7.123453452023678523, 17.78030770151605822 ) ) ;
#14790=CARTESIAN_POINT ( 'NONE',  ( 53.18981816583844591, 9.931948859054354983, 11.99999999999999645 ) ) ;
#14795=CARTESIAN_POINT ( 'NONE',  ( 51.46875000000000000, 6.999999999999992895, 13.75735931288071967 ) ) ;
#14797=CARTESIAN_POINT ( 'NONE',  ( 51.75000000000000711, 7.878679656440361612, 17.12132034355964549 ) ) ;
#14806=CARTESIAN_POINT ( 'NONE',  ( 56.34375000000000711, 8.757359312880723223, 18.00000000000000355 ) ) ;
#14822=CARTESIAN_POINT ( 'NONE',  ( 51.50231816583844591, 12.78030770151603868, 12.12345345202365188 ) ) ;
#14837=CARTESIAN_POINT ( 'NONE',  ( 56.62500000000000000, 12.82842712474620228, 17.82842712474617386 ) ) ;
#14843=CARTESIAN_POINT ( 'NONE',  ( 57.22106816583844591, 14.02818770551465377, 16.58880310854672757 ) ) ;
#14852=CARTESIAN_POINT ( 'NONE',  ( 54.90393183416157541, 14.02818770551463956, 13.41119689145323335 ) ) ;
#14898=CARTESIAN_POINT ( 'NONE',  ( 58.78125000000000711, 8.343145750507600766, 11.00000000000000533 ) ) ;
#14906=CARTESIAN_POINT ( 'NONE',  ( 53.34375000000000000, 8.757359312880723223, 18.00000000000000355 ) ) ;
#14915=CARTESIAN_POINT ( 'NONE',  ( 60.62268183416157541, 12.07320092032950676, 17.16943976678977180 ) ) ;
#14919=CARTESIAN_POINT ( 'NONE',  ( 53.34375000000000000, 8.757359312880723223, 18.00000000000000355 ) ) ;
#14931=CARTESIAN_POINT ( 'NONE',  ( 56.71875000000000711, 13.00000000000000711, 16.24264068711927322 ) ) ;
#14950=CARTESIAN_POINT ( 'NONE',  ( 58.72106816583844591, 13.02818770551464489, 16.17458954617363531 ) ) ;
#14964=CARTESIAN_POINT ( 'NONE',  ( 53.53125000000000000, 11.65685424949239923, 18.99999999999998934 ) ) ;
#14970=CARTESIAN_POINT ( 'NONE',  ( 54.59606816583844591, 11.58880310854672935, 10.97181229448534445 ) ) ;
#14980=CARTESIAN_POINT ( 'NONE',  ( 53.96643183416157541, 6.028187705514633343, 13.27509460956200016 ) ) ;
#14991=CARTESIAN_POINT ( 'NONE',  ( 53.53125000000000000, 11.24264068711929276, 18.00000000000000000 ) ) ;
#15022=CARTESIAN_POINT ( 'NONE',  ( 52.27893183416158251, 8.411196891453236901, 10.97181229448535511 ) ) ;
#15029=CARTESIAN_POINT ( 'NONE',  ( 52.78125000000000711, 8.757359312880703683, 11.99999999999999822 ) ) ;
#15035=CARTESIAN_POINT ( 'NONE',  ( 57.81018183416157541, 12.99999999999999822, 15.06805114094562192 ) ) ;
#15037=CARTESIAN_POINT ( 'NONE',  ( 55.59375000000000711, 11.24264068711927322, 11.99999999999998934 ) ) ;
#15044=CARTESIAN_POINT ( 'NONE',  ( 56.21643183416158251, 12.97181229448535689, 16.31069182806490758 ) ) ;
#15063=CARTESIAN_POINT ( 'NONE',  ( 51.12731816583844591, 12.87654654797634102, 17.78030770151602979 ) ) ;
#15084=CARTESIAN_POINT ( 'NONE',  ( 56.00231816583843170, 12.78030770151603868, 12.12345345202365188 ) ) ;
#15093=CARTESIAN_POINT ( 'NONE',  ( 59.43750000000000711, 10.00000000000001776, 18.99999999999999645 ) ) ;
#15134=CARTESIAN_POINT ( 'NONE',  ( 58.96875000000000711, 5.999999999999987566, 13.34314575050763452 ) ) ;
#15143=CARTESIAN_POINT ( 'NONE',  ( 56.71875000000000711, 13.00000000000000711, 16.24264068711927322 ) ) ;
#15151=CARTESIAN_POINT ( 'NONE',  ( 56.40393183416158251, 13.02818770551463778, 13.82541045382633982 ) ) ;
#15160=CARTESIAN_POINT ( 'NONE',  ( 55.46643183416158962, 7.028187705514638672, 13.68930817193508531 ) ) ;
#15180=CARTESIAN_POINT ( 'NONE',  ( 55.72106816583844591, 13.02818770551464489, 16.17458954617363531 ) ) ;
#15183=FACE_OUTER_BOUND ( 'NONE', #2522, .T. ) ;
#15204=CARTESIAN_POINT ( 'NONE',  ( 52.09143183416158251, 11.72490539043799984, 11.02818770551463246 ) ) ;
#15251=CARTESIAN_POINT ( 'NONE',  ( 52.09143183416158251, 11.72490539043799984, 11.02818770551463246 ) ) ;
#15261=CARTESIAN_POINT ( 'NONE',  ( 57.18750000000000000, 9.999999999999989342, 11.99999999999999467 ) ) ;
#15269=CARTESIAN_POINT ( 'NONE',  ( 57.34143183416159673, 8.689308171935088865, 17.97181229448535689 ) ) ;
#15280=CARTESIAN_POINT ( 'NONE',  ( 56.96643183416158251, 7.028187705514638672, 13.68930817193508531 ) ) ;
#15288=DIRECTION ( 'NONE',  ( -0.06805114094563445570, 0.7054675904022865707, 0.7054675904022728039 ) ) ;
#15302=CARTESIAN_POINT ( 'NONE',  ( 53.47106816583843880, 6.971812294485350670, 13.82541045382635403 ) ) ;
#15330=CARTESIAN_POINT ( 'NONE',  ( 58.03125000000000711, 11.65685424949239923, 18.99999999999998934 ) ) ;
#15374=CARTESIAN_POINT ( 'NONE',  ( 59.81250000000000711, 14.00000000000000000, 14.99999999999997691 ) ) ;
#15385=CARTESIAN_POINT ( 'NONE',  ( 58.31250000000000000, 13.00000000000000000, 14.99999999999998757 ) ) ;
#15391=CARTESIAN_POINT ( 'NONE',  ( 56.68518183416157541, 10.06805114094562548, 11.99999999999999645 ) ) ;
#15400=CARTESIAN_POINT ( 'NONE',  ( 59.40393183416158251, 13.02818770551463778, 13.82541045382633982 ) ) ;
#15420=CARTESIAN_POINT ( 'NONE',  ( 55.25231816583843170, 7.926799079670502124, 17.16943976678978245 ) ) ;
#15445=CARTESIAN_POINT ( 'NONE',  ( 55.50000000000000711, 12.82842712474617741, 12.17157287525379239 ) ) ;
#15495=CARTESIAN_POINT ( 'NONE',  ( 52.68750000000000711, 9.999999999999989342, 11.99999999999999467 ) ) ;
#15501=CARTESIAN_POINT ( 'NONE',  ( 55.18518183416157541, 10.06805114094562548, 11.99999999999999645 ) ) ;
#15512=CARTESIAN_POINT ( 'NONE',  ( 58.18518183416157541, 10.06805114094562548, 11.99999999999999645 ) ) ;
#15526=CARTESIAN_POINT ( 'NONE',  ( 54.97106816583843880, 6.971812294485350670, 13.82541045382635403 ) ) ;
#15536=CARTESIAN_POINT ( 'NONE',  ( 53.37731816583844591, 7.830560233210212218, 12.92679907967049679 ) ) ;
#15565=CARTESIAN_POINT ( 'NONE',  ( 57.46875000000000711, 5.999999999999987566, 13.34314575050763452 ) ) ;
#15568=CARTESIAN_POINT ( 'NONE',  ( 51.00000000000000711, 12.82842712474617741, 12.17157287525379239 ) ) ;
#15590=ORIENTED_EDGE ( 'NONE', *, *, #7596, .T. ) ;
#15615=CARTESIAN_POINT ( 'NONE',  ( 52.03124999999999289, 11.24264068711929276, 18.00000000000000355 ) ) ;
#15622=CARTESIAN_POINT ( 'NONE',  ( 59.96643183416158251, 6.028187705514633343, 13.27509460956200016 ) ) ;
#15633=CARTESIAN_POINT ( 'NONE',  ( 53.02893183416157541, 11.17458954617365663, 18.02818770551464311 ) ) ;
#15641=CARTESIAN_POINT ( 'NONE',  ( 50.18981816583844591, 9.931948859054346102, 10.99999999999999467 ) ) ;
#15654=CARTESIAN_POINT ( 'NONE',  ( 52.25231816583844591, 7.926799079670502124, 17.16943976678978245 ) ) ;
#15682=CARTESIAN_POINT ( 'NONE',  ( 56.43750000000000000, 10.00000000000001776, 18.99999999999999645 ) ) ;
#15735=CARTESIAN_POINT ( 'NONE',  ( 51.84375000000001421, 8.757359312880723223, 18.00000000000000355 ) ) ;
#15744=CARTESIAN_POINT ( 'NONE',  ( 52.37268183416157541, 7.926799079670491466, 12.83056023321021755 ) ) ;
#15753=CARTESIAN_POINT ( 'NONE',  ( 54.62268183416157541, 12.07320092032950676, 17.16943976678977180 ) ) ;
#15761=CARTESIAN_POINT ( 'NONE',  ( 57.68981816583843170, 9.931948859054354983, 11.99999999999999645 ) ) ;
#15767=CARTESIAN_POINT ( 'NONE',  ( 58.12500000000000000, 12.12132034355964727, 17.12132034355963484 ) ) ;
#15769=CARTESIAN_POINT ( 'NONE',  ( 59.62500000000000711, 12.12132034355964727, 17.12132034355963484 ) ) ;
#15784=DIRECTION ( 'NONE',  ( -0.000000000000000000, 0.000000000000000000, -1.000000000000000000 ) ) ;
#15793=CARTESIAN_POINT ( 'NONE',  ( 55.25231816583843170, 7.219692298483957771, 17.87654654797633924 ) ) ;
#15811=CARTESIAN_POINT ( 'NONE',  ( 53.34375000000000000, 8.343145750507638070, 19.00000000000000711 ) ) ;
#15849=CARTESIAN_POINT ( 'NONE',  ( 60.00000000000001421, 10.96484721591755473, 18.28038746411511184 ) ) ;
#15858=CARTESIAN_POINT ( 'NONE',  ( 53.59143183416158962, 11.31069182806491291, 12.02818770551463778 ) ) ;
#15869=CARTESIAN_POINT ( 'NONE',  ( 50.75231816583844591, 7.219692298483957771, 17.87654654797633924 ) ) ;
#15875=CARTESIAN_POINT ( 'NONE',  ( 58.50000000000000000, 12.12132034355963484, 12.87867965644034740 ) ) ;
#15877=CARTESIAN_POINT ( 'NONE',  ( 51.22106816583844591, 13.02818770551464489, 16.17458954617363531 ) ) ;
#15885=CARTESIAN_POINT ( 'NONE',  ( 58.40625000000000711, 12.99999999999999645, 13.75735931288070191 ) ) ;
#15902=CARTESIAN_POINT ( 'NONE',  ( 56.28356816583844591, 8.275094609561968184, 11.02818770551464667 ) ) ;
#15918=CARTESIAN_POINT ( 'NONE',  ( 58.15856816583844591, 6.028187705514649330, 16.72490539043803182 ) ) ;
#15935=CARTESIAN_POINT ( 'NONE',  ( 57.65625000000001421, 7.000000000000002665, 16.24264068711929099 ) ) ;
#15955=CARTESIAN_POINT ( 'NONE',  ( 60.00000000000000000, 11.41727695452472169, 17.97316538709347356 ) ) ;
#15966=CARTESIAN_POINT ( 'NONE',  ( 52.93518183416157541, 9.931948859054372747, 17.99999999999999645 ) ) ;
#15977=CARTESIAN_POINT ( 'NONE',  ( 50.37731816583844591, 7.123453452023657206, 12.21969229848395599 ) ) ;
#15986=CARTESIAN_POINT ( 'NONE',  ( 57.18750000000000000, 9.999999999999989342, 11.99999999999999467 ) ) ;
#15991=CARTESIAN_POINT ( 'NONE',  ( 56.71875000000000711, 13.00000000000000711, 16.24264068711927322 ) ) ;
#15999=CARTESIAN_POINT ( 'NONE',  ( 59.90625000000000711, 12.99999999999999645, 13.75735931288070191 ) ) ;
#16000=( NAMED_UNIT ( * ) SI_UNIT ( $, .STERADIAN. ) SOLID_ANGLE_UNIT ( ) );
#16019=CARTESIAN_POINT ( 'NONE',  ( 52.50000000000000711, 12.82842712474617741, 12.17157287525379239 ) ) ;
#16028=AXIS2_PLACEMENT_3D ( 'NONE', #16385, #16731, #11004 ) ;
#16040=CARTESIAN_POINT ( 'NONE',  ( 54.18750000000000711, 9.999999999999978684, 10.99999999999999645 ) ) ;
#16057=CARTESIAN_POINT ( 'NONE',  ( 59.81250000000000711, 13.00000000000000000, 14.99999999999998757 ) ) ;
#16081=CARTESIAN_POINT ( 'NONE',  ( 60.00000000000001421, 13.54696164955606008, 13.15578628297699382 ) ) ;
#16091=CARTESIAN_POINT ( 'NONE',  ( 59.49768183416157541, 12.87654654797631792, 12.21969229848393113 ) ) ;
#16096=ORIENTED_EDGE ( 'NONE', *, *, #21498, .T. ) ;
#16104=CARTESIAN_POINT ( 'NONE',  ( 50.56481816583844591, 6.999999999999998224, 15.06805114094563436 ) ) ;
#16110=CARTESIAN_POINT ( 'NONE',  ( 58.96875000000000711, 6.999999999999992895, 13.75735931288071967 ) ) ;
#16113=CARTESIAN_POINT ( 'NONE',  ( 59.53125000000000000, 11.24264068711929276, 18.00000000000000355 ) ) ;
#16141=CARTESIAN_POINT ( 'NONE',  ( 58.15856816583844591, 6.028187705514649330, 16.72490539043803182 ) ) ;
#16159=CARTESIAN_POINT ( 'NONE',  ( 52.50000000000000711, 12.82842712474617741, 12.17157287525379239 ) ) ;
#16167=CARTESIAN_POINT ( 'NONE',  ( 58.27893183416158962, 8.411196891453236901, 10.97181229448535511 ) ) ;
#16174=CARTESIAN_POINT ( 'NONE',  ( 58.12500000000000000, 12.12132034355964727, 17.12132034355963484 ) ) ;
#16194=CARTESIAN_POINT ( 'NONE',  ( 60.00000000000000000, 12.85334760243663155, 16.18560892438961929 ) ) ;
#16205=CARTESIAN_POINT ( 'NONE',  ( 55.74768183416157541, 7.123453452023678523, 17.78030770151605822 ) ) ;
#16215=CARTESIAN_POINT ( 'NONE',  ( 59.43750000000000711, 10.00000000000000711, 17.99999999999999645 ) ) ;
#16222=CARTESIAN_POINT ( 'NONE',  ( 55.03125000000000000, 11.24264068711929276, 18.00000000000000355 ) ) ;
#16224=CARTESIAN_POINT ( 'NONE',  ( 59.06250000000000711, 6.999999999999997335, 15.00000000000000533 ) ) ;
#16233=CARTESIAN_POINT ( 'NONE',  ( 53.25000000000000711, 7.878679656440361612, 17.12132034355964549 ) ) ;
#16253=CARTESIAN_POINT ( 'NONE',  ( 58.53356816583845301, 11.72490539043803004, 18.97181229448534268 ) ) ;
#16270=CARTESIAN_POINT ( 'NONE',  ( 58.50000000000000000, 12.82842712474617741, 12.17157287525379239 ) ) ;
#16274=CARTESIAN_POINT ( 'NONE',  ( 54.09375000000000711, 11.65685424949236193, 10.99999999999998401 ) ) ;
#16284=CARTESIAN_POINT ( 'NONE',  ( 59.77893183416158962, 8.411196891453236901, 10.97181229448535511 ) ) ;
#16293=CARTESIAN_POINT ( 'NONE',  ( 54.46875000000000000, 6.999999999999992006, 13.75735931288071967 ) ) ;
#16325=CARTESIAN_POINT ( 'NONE',  ( 56.40393183416158251, 14.02818770551463956, 13.41119689145323335 ) ) ;
#16331=CARTESIAN_POINT ( 'NONE',  ( 60.00000000000000711, 12.12132034355963484, 12.87867965644034740 ) ) ;
#16337=CARTESIAN_POINT ( 'NONE',  ( 60.52893183416158251, 11.17458954617365663, 18.02818770551464311 ) ) ;
#16339=CARTESIAN_POINT ( 'NONE',  ( 56.06250000000000000, 6.999999999999997335, 15.00000000000000533 ) ) ;
#16347=CARTESIAN_POINT ( 'NONE',  ( 54.93750000000000711, 10.00000000000000711, 17.99999999999999645 ) ) ;
#16367=CARTESIAN_POINT ( 'NONE',  ( 54.31481816583844591, 14.00000000000000178, 14.93194885905434610 ) ) ;
#16383=CARTESIAN_POINT ( 'NONE',  ( 57.84375000000000711, 8.343145750507636293, 19.00000000000000000 ) ) ;
#16385=CARTESIAN_POINT ( 'NONE',  ( 51.00000000000000711, 12.47487373415290612, 12.52512626584706901 ) ) ;
#16387=CARTESIAN_POINT ( 'NONE',  ( 56.93981816583843170, 10.06805114094564857, 19.00000000000000000 ) ) ;
#16390=DIRECTION ( 'NONE',  ( 0.000000000000000000, -0.7071067811865414665, 0.7071067811865536790 ) ) ;
#16397=CARTESIAN_POINT ( 'NONE',  ( 60.43518183416157541, 9.931948859054379852, 18.99999999999999289 ) ) ;
#16404=CARTESIAN_POINT ( 'NONE',  ( 57.75000000000000000, 7.878679656440361612, 17.12132034355964549 ) ) ;
#16439=CARTESIAN_POINT ( 'NONE',  ( 54.06018183416157541, 5.999999999999996447, 14.93194885905437808 ) ) ;
#16450=CARTESIAN_POINT ( 'NONE',  ( 51.87731816583844591, 7.830560233210212218, 12.92679907967049679 ) ) ;
#16457=CARTESIAN_POINT ( 'NONE',  ( 55.21875000000000000, 13.00000000000000711, 16.24264068711927322 ) ) ;
#16460=CARTESIAN_POINT ( 'NONE',  ( 51.18750000000000711, 9.999999999999989342, 11.99999999999999467 ) ) ;
#16467=CARTESIAN_POINT ( 'NONE',  ( 56.25000000000000711, 7.878679656440361612, 17.12132034355964549 ) ) ;
#16486=CARTESIAN_POINT ( 'NONE',  ( 53.93981816583844591, 10.06805114094564857, 19.00000000000000000 ) ) ;
#16500=CARTESIAN_POINT ( 'NONE',  ( 53.71875000000000711, 14.00000000000001066, 16.65685424949235482 ) ) ;
#16503=CARTESIAN_POINT ( 'NONE',  ( 51.87731816583844591, 7.123453452023657206, 12.21969229848395599 ) ) ;
#16514=CARTESIAN_POINT ( 'NONE',  ( 53.77893183416158251, 8.411196891453236901, 10.97181229448535511 ) ) ;
#16521=CARTESIAN_POINT ( 'NONE',  ( 53.90625000000000000, 12.99999999999999645, 13.75735931288070191 ) ) ;
#16556=CARTESIAN_POINT ( 'NONE',  ( 57.15393183416157541, 5.971812294485358663, 16.58880310854675599 ) ) ;
#16562=CARTESIAN_POINT ( 'NONE',  ( 51.03356816583844591, 11.31069182806492712, 17.97181229448534623 ) ) ;
#16568=CARTESIAN_POINT ( 'NONE',  ( 60.34143183416158962, 8.689308171935088865, 17.97181229448535689 ) ) ;
#16572=CARTESIAN_POINT ( 'NONE',  ( 53.81250000000000711, 13.00000000000000000, 14.99999999999998757 ) ) ;
#16580=CARTESIAN_POINT ( 'NONE',  ( 51.46875000000000000, 6.999999999999992895, 13.75735931288071967 ) ) ;
#16598=CARTESIAN_POINT ( 'NONE',  ( 51.59606816583843170, 11.58880310854672935, 10.97181229448534445 ) ) ;
#16613=CARTESIAN_POINT ( 'NONE',  ( 57.65625000000001421, 6.000000000000004441, 16.65685424949239390 ) ) ;
#16617=CARTESIAN_POINT ( 'NONE',  ( 56.37731816583843170, 7.123453452023657206, 12.21969229848395599 ) ) ;
#16626=CARTESIAN_POINT ( 'NONE',  ( 54.06018183416157541, 5.999999999999996447, 14.93194885905437808 ) ) ;
#16670=CARTESIAN_POINT ( 'NONE',  ( 58.18518183416157541, 10.06805114094561659, 10.99999999999999645 ) ) ;
#16681=CARTESIAN_POINT ( 'NONE',  ( 53.53125000000000000, 11.24264068711929276, 18.00000000000000355 ) ) ;
#16688=CARTESIAN_POINT ( 'NONE',  ( 60.06018183416157541, 7.000000000000000000, 14.93194885905437097 ) ) ;
#16693=VERTEX_POINT ( 'NONE', #21225 ) ;
#16697=CARTESIAN_POINT ( 'NONE',  ( 57.18750000000000000, 9.999999999999989342, 11.99999999999999467 ) ) ;
#16714=CARTESIAN_POINT ( 'NONE',  ( 52.72106816583844591, 14.02818770551465377, 16.58880310854672757 ) ) ;
#16729=CARTESIAN_POINT ( 'NONE',  ( 54.46875000000000000, 5.999999999999987566, 13.34314575050763452 ) ) ;
#16731=DIRECTION ( 'NONE',  ( 0.06805114094563399774, -0.7054675904022866817, -0.7054675904022729149 ) ) ;
#16735=CARTESIAN_POINT ( 'NONE',  ( 52.06481816583844591, 5.999999999999996447, 15.06805114094564502 ) ) ;
#16745=CARTESIAN_POINT ( 'NONE',  ( 53.87268183416157541, 7.219692298483935566, 12.12345345202367675 ) ) ;
#16755=CARTESIAN_POINT ( 'NONE',  ( 53.81250000000000711, 13.00000000000000000, 14.99999999999998757 ) ) ;
#16770=AXIS2_PLACEMENT_3D ( 'NONE', #13870, #21128, #15784 ) ;
#16792=CARTESIAN_POINT ( 'NONE',  ( 59.62500000000000711, 12.82842712474620228, 17.82842712474617386 ) ) ;
#16802=CARTESIAN_POINT ( 'NONE',  ( 53.62500000000000711, 12.12132034355964727, 17.12132034355963484 ) ) ;
#16811=CARTESIAN_POINT ( 'NONE',  ( 56.02893183416158962, 11.17458954617365663, 18.02818770551464311 ) ) ;
#16814=CARTESIAN_POINT ( 'NONE',  ( 52.59375000000000711, 11.24264068711927322, 11.99999999999998934 ) ) ;
#16825=CARTESIAN_POINT ( 'NONE',  ( 56.59143183416158962, 11.31069182806491291, 12.02818770551463778 ) ) ;
#16843=CARTESIAN_POINT ( 'NONE',  ( 54.12731816583844591, 12.87654654797634102, 17.78030770151602979 ) ) ;
#16865=CARTESIAN_POINT ( 'NONE',  ( 53.37731816583844591, 7.123453452023657206, 12.21969229848395599 ) ) ;
#16873=CARTESIAN_POINT ( 'NONE',  ( 54.52893183416158962, 11.58880310854676132, 19.02818770551463956 ) ) ;
#16882=CARTESIAN_POINT ( 'NONE',  ( 53.15625000000000711, 7.000000000000002665, 16.24264068711929099 ) ) ;
#16916=CARTESIAN_POINT ( 'NONE',  ( 58.59375000000000711, 11.65685424949236193, 10.99999999999998401 ) ) ;
#16924=CARTESIAN_POINT ( 'NONE',  ( 55.40625000000000000, 12.99999999999999645, 13.75735931288070191 ) ) ;
#16931=CARTESIAN_POINT ( 'NONE',  ( 57.71643183416158251, 12.97181229448535689, 16.31069182806490758 ) ) ;
#16940=CARTESIAN_POINT ( 'NONE',  ( 58.84143183416158962, 8.689308171935088865, 17.97181229448535689 ) ) ;
#16957=CARTESIAN_POINT ( 'NONE',  ( 57.78356816583844591, 8.689308171935074654, 12.02818770551464489 ) ) ;
#16988=CARTESIAN_POINT ( 'NONE',  ( 55.46643183416158962, 6.028187705514633343, 13.27509460956200016 ) ) ;
#16996=CARTESIAN_POINT ( 'NONE',  ( 51.56250000000000711, 6.999999999999997335, 15.00000000000000533 ) ) ;
#17030=CARTESIAN_POINT ( 'NONE',  ( 55.78125000000000000, 8.343145750507600766, 11.00000000000000533 ) ) ;
#17038=CARTESIAN_POINT ( 'NONE',  ( 57.65625000000002132, 7.000000000000003553, 16.24264068711929099 ) ) ;
#17047=CARTESIAN_POINT ( 'NONE',  ( 54.34143183416158251, 8.689308171935088865, 17.97181229448535689 ) ) ;
#17056=CARTESIAN_POINT ( 'NONE',  ( 59.12268183416157541, 12.07320092032950676, 17.16943976678977180 ) ) ;
#17075=CARTESIAN_POINT ( 'NONE',  ( 54.22106816583844591, 13.02818770551464489, 16.17458954617363531 ) ) ;
#17098=CARTESIAN_POINT ( 'NONE',  ( 55.78125000000000000, 8.343145750507600766, 11.00000000000000533 ) ) ;
#17149=CARTESIAN_POINT ( 'NONE',  ( 59.34375000000000711, 8.343145750507638070, 19.00000000000000711 ) ) ;
#17159=CARTESIAN_POINT ( 'NONE',  ( 56.62500000000000000, 12.12132034355964727, 17.12132034355963484 ) ) ;
#17165=CARTESIAN_POINT ( 'NONE',  ( 58.37268183416157541, 7.926799079670491466, 12.83056023321021755 ) ) ;
#17176=CARTESIAN_POINT ( 'NONE',  ( 60.90393183416158962, 13.02818770551463778, 13.82541045382633982 ) ) ;
#17200=CARTESIAN_POINT ( 'NONE',  ( 54.03356816583844591, 11.31069182806492712, 17.97181229448534623 ) ) ;
#17217=CARTESIAN_POINT ( 'NONE',  ( 51.09375000000000711, 11.65685424949236015, 10.99999999999998579 ) ) ;
#17221=UNCERTAINTY_MEASURE_WITH_UNIT (LENGTH_MEASURE( 1.000000000000000082E-05 ), #19944, 'distance_accuracy_value', 'NONE');
#17229=CARTESIAN_POINT ( 'NONE',  ( 57.28125000000000711, 8.343145750507600766, 11.00000000000000533 ) ) ;
#17231=DIRECTION ( 'NONE',  ( 0.000000000000000000, 0.7071067811865414665, -0.7071067811865536790 ) ) ;
#17289=CARTESIAN_POINT ( 'NONE',  ( 58.09143183416158962, 11.31069182806491291, 12.02818770551463778 ) ) ;
#17299=CARTESIAN_POINT ( 'NONE',  ( 59.02893183416158251, 11.17458954617365663, 18.02818770551464311 ) ) ;
#17308=CARTESIAN_POINT ( 'NONE',  ( 57.78356816583844591, 8.689308171935074654, 12.02818770551464489 ) ) ;
#17319=CARTESIAN_POINT ( 'NONE',  ( 52.90856816583843880, 12.97181229448534978, 13.68930817193506755 ) ) ;
#17334=CARTESIAN_POINT ( 'NONE',  ( 51.93750000000000711, 10.00000000000001776, 18.99999999999999645 ) ) ;
#17344=CARTESIAN_POINT ( 'NONE',  ( 56.34375000000000711, 8.343145750507638070, 19.00000000000000711 ) ) ;
#17395=CARTESIAN_POINT ( 'NONE',  ( 51.93750000000000711, 10.00000000000000711, 17.99999999999999645 ) ) ;
#17397=AXIS2_PLACEMENT_3D ( 'NONE', #15568, #8011, #17231 ) ;
#17403=CARTESIAN_POINT ( 'NONE',  ( 53.40393183416157541, 13.02818770551463778, 13.82541045382633982 ) ) ;
#17413=CARTESIAN_POINT ( 'NONE',  ( 58.74768183416157541, 7.123453452023678523, 17.78030770151605822 ) ) ;
#17426=CARTESIAN_POINT ( 'NONE',  ( 57.12731816583843170, 12.16943976678978601, 17.07320092032949432 ) ) ;
#17437=CARTESIAN_POINT ( 'NONE',  ( 54.59606816583844591, 11.17458954617364242, 11.97181229448534800 ) ) ;
#17447=CARTESIAN_POINT ( 'NONE',  ( 59.71875000000000711, 13.00000000000000711, 16.24264068711927322 ) ) ;
#17465=CARTESIAN_POINT ( 'NONE',  ( 58.31250000000000000, 14.00000000000000000, 14.99999999999997691 ) ) ;
#17519=CARTESIAN_POINT ( 'NONE',  ( 53.31018183416157541, 12.99999999999999822, 15.06805114094562192 ) ) ;
#17532=CARTESIAN_POINT ( 'NONE',  ( 53.96643183416157541, 7.028187705514638672, 13.68930817193508531 ) ) ;
#17539=CARTESIAN_POINT ( 'NONE',  ( 56.56481816583843170, 6.999999999999998224, 15.06805114094563436 ) ) ;
#17551=CARTESIAN_POINT ( 'NONE',  ( 60.00000000000000711, 12.12132034355963484, 12.87867965644034740 ) ) ;
#17554=CARTESIAN_POINT ( 'NONE',  ( 50.28356816583843880, 8.689308171935074654, 12.02818770551464489 ) ) ;
#17560=ORIENTED_EDGE ( 'NONE', *, *, #9539, .F. ) ;
#17564=PRESENTATION_STYLE_ASSIGNMENT (( #21005 ) ) ;
#17582=CARTESIAN_POINT ( 'NONE',  ( 53.25000000000000711, 7.171572875253819923, 17.82842712474619873 ) ) ;
#17644=CARTESIAN_POINT ( 'NONE',  ( 60.00000000000001421, 13.96345569325843172, 15.23269126663819506 ) ) ;
#17654=CARTESIAN_POINT ( 'NONE',  ( 60.15393183416158962, 5.971812294485358663, 16.58880310854675599 ) ) ;
#17662=CARTESIAN_POINT ( 'NONE',  ( 55.15856816583844591, 7.028187705514647554, 16.31069182806492179 ) ) ;
#17670=CARTESIAN_POINT ( 'NONE',  ( 57.37500000000000000, 7.878679656440349177, 12.87867965644035984 ) ) ;
#17687=UNCERTAINTY_MEASURE_WITH_UNIT (LENGTH_MEASURE( 1.000000000000000082E-05 ), #19455, 'distance_accuracy_value', 'NONE');
#17689=EDGE_CURVE ( 'NONE', #8676, #1478, #9409, .T. ) ;
#17696=CARTESIAN_POINT ( 'NONE',  ( 55.53356816583845301, 11.72490539043803004, 18.97181229448534268 ) ) ;
#17714=CARTESIAN_POINT ( 'NONE',  ( 54.46875000000000000, 5.999999999999987566, 13.34314575050763452 ) ) ;
#17731=CARTESIAN_POINT ( 'NONE',  ( 59.34375000000000711, 8.757359312880723223, 18.00000000000000711 ) ) ;
#17741=CLOSED_SHELL ( 'NONE', ( #608, #22380, #12591, #4241, #7770 ) ) ;
#17751=CARTESIAN_POINT ( 'NONE',  ( 59.99999999999182876, 10.99015334700498236, 18.43425161108635280 ) ) ;
#17760=CARTESIAN_POINT ( 'NONE',  ( 59.12268183416157541, 12.78030770151606177, 17.87654654797631792 ) ) ;
#17770=CARTESIAN_POINT ( 'NONE',  ( 54.68981816583844591, 9.931948859054354983, 11.99999999999999645 ) ) ;
#17779=CARTESIAN_POINT ( 'NONE',  ( 56.81250000000000000, 13.00000000000000000, 14.99999999999998757 ) ) ;
#17788=CARTESIAN_POINT ( 'NONE',  ( 58.78125000000000711, 8.757359312880703683, 11.99999999999999822 ) ) ;
#17790=( NAMED_UNIT ( * ) PLANE_ANGLE_UNIT ( ) SI_UNIT ( $, .RADIAN. ) );
#17807=CARTESIAN_POINT ( 'NONE',  ( 52.78125000000000711, 8.343145750507600766, 11.00000000000000533 ) ) ;
#17821=CARTESIAN_POINT ( 'NONE',  ( 59.43750000000000711, 10.00000000000001776, 18.99999999999999645 ) ) ;
#17825=CARTESIAN_POINT ( 'NONE',  ( 55.12500000000000711, 12.82842712474620228, 17.82842712474617386 ) ) ;
#17841=CARTESIAN_POINT ( 'NONE',  ( 55.59375000000002132, 11.24264068711927322, 11.99999999999998934 ) ) ;
#17843=DIRECTION ( 'NONE',  ( 1.000000000000000000, 0.000000000000000000, 0.000000000000000000 ) ) ;
#17863=CARTESIAN_POINT ( 'NONE',  ( 60.00000000000000711, 13.77581299381601099, 16.13248257417277642 ) ) ;
#17876=CARTESIAN_POINT ( 'NONE',  ( 58.93518183416157541, 9.931948859054379852, 18.99999999999999289 ) ) ;
#17884=CARTESIAN_POINT ( 'NONE',  ( 51.31481816583844591, 12.99999999999999822, 14.93194885905435676 ) ) ;
#17891=CARTESIAN_POINT ( 'NONE',  ( 56.53125000000000711, 11.24264068711929276, 18.00000000000000355 ) ) ;
#17895=CARTESIAN_POINT ( 'NONE',  ( 51.78356816583844591, 8.689308171935074654, 12.02818770551464489 ) ) ;
#17901=ORIENTED_EDGE ( 'NONE', *, *, #21498, .F. ) ;
#17922=CARTESIAN_POINT ( 'NONE',  ( 58.62731816583843170, 12.87654654797634102, 17.78030770151602979 ) ) ;
#17942=CARTESIAN_POINT ( 'NONE',  ( 51.75000000000000711, 7.171572875253819923, 17.82842712474619873 ) ) ;
#17951=CARTESIAN_POINT ( 'NONE',  ( 57.43518183416157541, 9.931948859054379852, 18.99999999999999289 ) ) ;
#17960=CARTESIAN_POINT ( 'NONE',  ( 57.09375000000000711, 11.24264068711927322, 11.99999999999998934 ) ) ;
#17995=CARTESIAN_POINT ( 'NONE',  ( 54.43518183416157541, 9.931948859054379852, 18.99999999999999289 ) ) ;
#18007=CARTESIAN_POINT ( 'NONE',  ( 59.71875000000000711, 13.00000000000000711, 16.24264068711927322 ) ) ;
#18017=CARTESIAN_POINT ( 'NONE',  ( 50.84606816583843880, 8.825410453826357582, 18.02818770551464667 ) ) ;
#18025=CARTESIAN_POINT ( 'NONE',  ( 53.71875000000002132, 13.00000000000000711, 16.24264068711927322 ) ) ;
#18044=CARTESIAN_POINT ( 'NONE',  ( 56.75231816583843170, 7.219692298483957771, 17.87654654797633924 ) ) ;
#18061=CARTESIAN_POINT ( 'NONE',  ( 55.21875000000000000, 14.00000000000000888, 16.65685424949235482 ) ) ;
#18070=CARTESIAN_POINT ( 'NONE',  ( 60.81018183416157541, 14.00000000000000000, 15.06805114094561304 ) ) ;
#18077=CARTESIAN_POINT ( 'NONE',  ( 57.93750000000000000, 10.00000000000000711, 17.99999999999999645 ) ) ;
#18108=CARTESIAN_POINT ( 'NONE',  ( 53.02893183416157541, 11.58880310854676132, 19.02818770551463956 ) ) ;
#18119=CARTESIAN_POINT ( 'NONE',  ( 58.96875000000000711, 6.999999999999992895, 13.75735931288071967 ) ) ;
#18124=CARTESIAN_POINT ( 'NONE',  ( 54.75000000000000711, 7.878679656440361612, 17.12132034355964549 ) ) ;
#18127=CARTESIAN_POINT ( 'NONE',  ( 55.96875000000000000, 6.999999999999992895, 13.75735931288071967 ) ) ;
#18135=CARTESIAN_POINT ( 'NONE',  ( 55.03125000000000000, 11.24264068711929276, 18.00000000000000355 ) ) ;
#18153=CARTESIAN_POINT ( 'NONE',  ( 55.62731816583843170, 12.87654654797634102, 17.78030770151602979 ) ) ;
#18170=CARTESIAN_POINT ( 'NONE',  ( 56.06250000000000000, 5.999999999999996447, 15.00000000000001599 ) ) ;
#18174=CARTESIAN_POINT ( 'NONE',  ( 54.37500000000000711, 7.171572875253794166, 12.17157287525381726 ) ) ;
#18185=CARTESIAN_POINT ( 'NONE',  ( 58.56018183416157541, 5.999999999999996447, 14.93194885905437808 ) ) ;
#18190=EDGE_LOOP ( 'NONE', ( #13871, #15590, #16096, #14228 ) ) ;
#18192=CARTESIAN_POINT ( 'NONE',  ( 55.68750000000000000, 9.999999999999989342, 11.99999999999999467 ) ) ;
#18223=CARTESIAN_POINT ( 'NONE',  ( 55.84143183416158251, 8.275094609562001935, 18.97181229448536044 ) ) ;
#18230=CARTESIAN_POINT ( 'NONE',  ( 52.72106816583844591, 13.02818770551464489, 16.17458954617363531 ) ) ;
#18237=CARTESIAN_POINT ( 'NONE',  ( 53.34375000000000000, 8.757359312880723223, 18.00000000000000355 ) ) ;
#18239=CARTESIAN_POINT ( 'NONE',  ( 51.46875000000000000, 6.999999999999992895, 13.75735931288071967 ) ) ;
#18246=CARTESIAN_POINT ( 'NONE',  ( 55.68750000000000000, 9.999999999999989342, 11.99999999999999467 ) ) ;
#18266=CARTESIAN_POINT ( 'NONE',  ( 51.40856816583843880, 13.97181229448534978, 13.27509460956196641 ) ) ;
#18284=CARTESIAN_POINT ( 'NONE',  ( 53.81250000000000711, 14.00000000000000000, 14.99999999999997691 ) ) ;
#18288=CARTESIAN_POINT ( 'NONE',  ( 57.12731816583843170, 12.87654654797634102, 17.78030770151602979 ) ) ;
#18303=CARTESIAN_POINT ( 'NONE',  ( 53.68518183416157541, 10.06805114094561659, 10.99999999999999645 ) ) ;
#18310=CARTESIAN_POINT ( 'NONE',  ( 51.18750000000000711, 9.999999999999989342, 11.99999999999999467 ) ) ;
#18347=CARTESIAN_POINT ( 'NONE',  ( 54.24768183416157541, 7.123453452023678523, 17.78030770151605822 ) ) ;
#18355=CARTESIAN_POINT ( 'NONE',  ( 52.43981816583844591, 10.06805114094563791, 17.99999999999999645 ) ) ;
#18362=CARTESIAN_POINT ( 'NONE',  ( 60.99768183416157541, 12.16943976678977535, 12.92679907967048614 ) ) ;
#18365=CARTESIAN_POINT ( 'NONE',  ( 54.84375000000000000, 8.757359312880723223, 18.00000000000000355 ) ) ;
#18372=CARTESIAN_POINT ( 'NONE',  ( 53.06250000000000711, 6.999999999999997335, 15.00000000000000533 ) ) ;
#18388=CARTESIAN_POINT ( 'NONE',  ( 54.68981816583844591, 9.931948859054346102, 10.99999999999999467 ) ) ;
#18405=CARTESIAN_POINT ( 'NONE',  ( 58.21875000000000711, 14.00000000000001066, 16.65685424949235482 ) ) ;
#18409=CARTESIAN_POINT ( 'NONE',  ( 56.28356816583844591, 8.275094609561968184, 11.02818770551464667 ) ) ;
#18416=CARTESIAN_POINT ( 'NONE',  ( 59.71875000000000711, 14.00000000000000888, 16.65685424949235482 ) ) ;
#18425=CARTESIAN_POINT ( 'NONE',  ( 54.00000000000000711, 12.12132034355963484, 12.87867965644034740 ) ) ;
#18460=CARTESIAN_POINT ( 'NONE',  ( 54.52893183416158962, 11.58880310854676132, 19.02818770551463956 ) ) ;
#18469=CARTESIAN_POINT ( 'NONE',  ( 54.09375000000000711, 11.24264068711927322, 11.99999999999998934 ) ) ;
#18474=CARTESIAN_POINT ( 'NONE',  ( 52.50000000000000711, 12.12132034355963484, 12.87867965644034740 ) ) ;
#18476=CARTESIAN_POINT ( 'NONE',  ( 52.21875000000002842, 13.00000000000000711, 16.24264068711927322 ) ) ;
#18483=CARTESIAN_POINT ( 'NONE',  ( 57.09375000000000711, 11.24264068711927322, 11.99999999999998934 ) ) ;
#18499=CARTESIAN_POINT ( 'NONE',  ( 54.40856816583843880, 13.97181229448534978, 13.27509460956196641 ) ) ;
#18513=CARTESIAN_POINT ( 'NONE',  ( 54.84375000000000711, 8.343145750507636293, 19.00000000000000000 ) ) ;
#18517=CARTESIAN_POINT ( 'NONE',  ( 55.25231816583843170, 7.219692298483957771, 17.87654654797633924 ) ) ;
#18527=CARTESIAN_POINT ( 'NONE',  ( 55.09143183416158962, 11.72490539043799984, 11.02818770551463246 ) ) ;
#18575=CARTESIAN_POINT ( 'NONE',  ( 59.71875000000000711, 14.00000000000000888, 16.65685424949235482 ) ) ;
#18585=CARTESIAN_POINT ( 'NONE',  ( 54.46875000000000000, 6.999999999999992895, 13.75735931288071967 ) ) ;
#18594=CARTESIAN_POINT ( 'NONE',  ( 59.49768183416157541, 12.16943976678977535, 12.92679907967048614 ) ) ;
#18596=CARTESIAN_POINT ( 'NONE',  ( 55.31250000000000711, 13.00000000000000000, 14.99999999999998757 ) ) ;
#18604=CARTESIAN_POINT ( 'NONE',  ( 60.52893183416158251, 11.17458954617365663, 18.02818770551464311 ) ) ;
#18621=CARTESIAN_POINT ( 'NONE',  ( 58.25231816583843170, 7.926799079670502124, 17.16943976678978245 ) ) ;
#18624=( NAMED_UNIT ( * ) PLANE_ANGLE_UNIT ( ) SI_UNIT ( $, .RADIAN. ) );
#18626=( BOUNDED_CURVE ( )  B_SPLINE_CURVE ( 2, ( #12244, #1295, #16057, #7070, #10804, #1540, #23213, #17731, #5383, #3109, #8881, #19974, #12722, #23584, #3577, #9116, #13389, #10684, #12478, #21413, #16174, #14147, #18077, #12360, #16404, #15935, #19742, #5140, #23462, #14269, #10450, #17960, #3342, #19512, #5029, #1658, #23347, #1774, #7321, #10912, #10569, #8750, #3219, #14387, #21649, #19622, #18192, #17841, #5259, #14626, #8632, #21886, #21531, #6954, #12602, #19863, #1410, #3466, #9000, #16293, #7194, #14509, #21773, #7782, #18425, #16521, #16755, #13294, #13067, #14991, #22241, #5496, #97, #16882, #7895, #20441, #12828, #5849, #568, #20206, #9589, #5971, #2002, #12942, #9457, #13178, #20087, #11027, #4051, #22357, #16996, #3686, #3815, #9237, #18310, #1893, #11380 ),
 .UNSPECIFIED., .F., .F. ) 
 B_SPLINE_CURVE_WITH_KNOTS ( ( 3, 2, 2, 2, 2, 2, 2, 2, 2, 2, 2, 2, 2, 2, 2, 2, 2, 2, 2, 2, 2, 2, 2, 2, 2, 2, 2, 2, 2, 2, 2, 2, 2, 2, 2, 2, 2, 2, 2, 2, 2, 2, 2, 2, 2, 2, 2, 2, 3 ),
 ( 0.000000000000000000, 0.02083333333333333218, 0.04166666666666666435, 0.06250000000000000000, 0.08333333333333332871, 0.1041666666666666713, 0.1250000000000000000, 0.1458333333333333426, 0.1666666666666666574, 0.1875000000000000000, 0.2083333333333333426, 0.2291666666666666574, 0.2500000000000000000, 0.2708333333333333148, 0.2916666666666666852, 0.3125000000000000000, 0.3333333333333333148, 0.3541666666666666852, 0.3750000000000000000, 0.3958333333333333148, 0.4166666666666666852, 0.4375000000000000000, 0.4583333333333333148, 0.4791666666666666852, 0.5000000000000000000, 0.5208333333333333703, 0.5416666666666666297, 0.5625000000000000000, 0.5833333333333333703, 0.6041666666666666297, 0.6250000000000000000, 0.6458333333333333703, 0.6666666666666666297, 0.6875000000000000000, 0.7083333333333333703, 0.7291666666666666297, 0.7500000000000000000, 0.7708333333333333703, 0.7916666666666666297, 0.8125000000000000000, 0.8333333333333333703, 0.8541666666666666297, 0.8750000000000000000, 0.8958333333333333703, 0.9166666666666666297, 0.9375000000000000000, 0.9583333333333333703, 0.9791666666666666297, 1.000000000000000000 ),
 .UNSPECIFIED. ) 
 CURVE ( )  GEOMETRIC_REPRESENTATION_ITEM ( )  RATIONAL_B_SPLINE_CURVE ( ( 1.000000000000000000, 0.9238795325112867385, 1.000000000000000000, 0.9238795325112867385, 1.000000000000000000, 0.9238795325112867385, 1.000000000000000000, 0.9238795325112867385, 1.000000000000000000, 0.9238795325112867385, 1.000000000000000000, 0.9238795325112867385, 1.000000000000000000, 0.9238795325112867385, 1.000000000000000000, 0.9238795325112867385, 1.000000000000000000, 0.9238795325112867385, 1.000000000000000000, 0.9238795325112867385, 1.000000000000000000, 0.9238795325112867385, 1.000000000000000000, 0.9238795325112867385, 1.000000000000000000, 0.9238795325112867385, 1.000000000000000000, 0.9238795325112867385, 1.000000000000000000, 0.9238795325112867385, 1.000000000000000000, 0.9238795325112867385, 1.000000000000000000, 0.9238795325112867385, 1.000000000000000000, 0.9238795325112867385, 1.000000000000000000, 0.9238795325112867385, 1.000000000000000000, 0.9238795325112867385, 1.000000000000000000, 0.9238795325112867385, 1.000000000000000000, 0.9238795325112867385, 1.000000000000000000, 0.9238795325112867385, 1.000000000000000000, 0.9238795325112867385, 1.000000000000000000, 0.9238795325112867385, 1.000000000000000000, 0.9238795325112867385, 1.000000000000000000, 0.9238795325112867385, 1.000000000000000000, 0.9238795325112867385, 1.000000000000000000, 0.9238795325112867385, 1.000000000000000000, 0.9238795325112867385, 1.000000000000000000, 0.9238795325112867385, 1.000000000000000000, 0.9238795325112867385, 1.000000000000000000, 0.9238795325112867385, 1.000000000000000000, 0.9238795325112867385, 1.000000000000000000, 0.9238795325112867385, 1.000000000000000000, 0.9238795325112867385, 1.000000000000000000, 0.9238795325112867385, 1.000000000000000000, 0.9238795325112867385, 1.000000000000000000, 0.9238795325112867385, 1.000000000000000000, 0.9238795325112867385, 1.000000000000000000, 0.9238795325112867385, 1.000000000000000000, 0.9238795325112867385, 1.000000000000000000, 0.9238795325112867385, 1.000000000000000000, 0.9238795325112867385, 1.000000000000000000, 0.9238795325112867385, 1.000000000000000000, 0.9238795325112867385, 1.000000000000000000, 0.9238795325112867385, 1.000000000000000000, 0.9238795325112867385, 1.000000000000000000 ) ) 
 REPRESENTATION_ITEM ( '' )  );
#18637=CARTESIAN_POINT ( 'NONE',  ( 58.03125000000000711, 11.65685424949239923, 18.99999999999998934 ) ) ;
#18643=CARTESIAN_POINT ( 'NONE',  ( 57.31481816583843170, 14.00000000000000178, 14.93194885905434610 ) ) ;
#18651=CARTESIAN_POINT ( 'NONE',  ( 51.99768183416157541, 12.87654654797631792, 12.21969229848393113 ) ) ;
#18697=CARTESIAN_POINT ( 'NONE',  ( 59.06250000000000711, 5.999999999999996447, 15.00000000000001599 ) ) ;
#18708=CARTESIAN_POINT ( 'NONE',  ( 57.28125000000000711, 8.757359312880703683, 11.99999999999999822 ) ) ;
#18716=CARTESIAN_POINT ( 'NONE',  ( 56.49768183416158962, 12.16943976678977535, 12.92679907967048614 ) ) ;
#18727=CARTESIAN_POINT ( 'NONE',  ( 56.40393183416158251, 13.02818770551463778, 13.82541045382633982 ) ) ;
#18750=CARTESIAN_POINT ( 'NONE',  ( 53.28356816583845301, 8.275094609561968184, 11.02818770551464667 ) ) ;
#18753=CARTESIAN_POINT ( 'NONE',  ( 60.00000000000000711, 12.82842712474617741, 12.17157287525379239 ) ) ;
#18770=CARTESIAN_POINT ( 'NONE',  ( 53.93981816583844591, 10.06805114094564857, 19.00000000000000000 ) ) ;
#18779=CARTESIAN_POINT ( 'NONE',  ( 55.18518183416157541, 10.06805114094561659, 10.99999999999999645 ) ) ;
#18783=DIRECTION ( 'NONE',  ( 0.000000000000000000, -0.7071067811865406894, 0.7071067811865545671 ) ) ;
#18818=CARTESIAN_POINT ( 'NONE',  ( 57.65625000000002132, 6.000000000000004441, 16.65685424949239390 ) ) ;
#18826=CARTESIAN_POINT ( 'NONE',  ( 55.59375000000000711, 11.24264068711927322, 11.99999999999998934 ) ) ;
#18832=CARTESIAN_POINT ( 'NONE',  ( 56.12268183416157541, 12.07320092032950676, 17.16943976678977180 ) ) ;
#18842=CARTESIAN_POINT ( 'NONE',  ( 58.56018183416157541, 7.000000000000000000, 14.93194885905437097 ) ) ;
#18859=CARTESIAN_POINT ( 'NONE',  ( 58.15856816583844591, 7.028187705514647554, 16.31069182806492179 ) ) ;
#18886=CARTESIAN_POINT ( 'NONE',  ( 53.71875000000002132, 14.00000000000000888, 16.65685424949235482 ) ) ;
#18932=CARTESIAN_POINT ( 'NONE',  ( 52.37268183416157541, 7.219692298483935566, 12.12345345202367675 ) ) ;
#18940=CARTESIAN_POINT ( 'NONE',  ( 58.21875000000000711, 13.00000000000000711, 16.24264068711927322 ) ) ;
#18946=CARTESIAN_POINT ( 'NONE',  ( 58.93518183416157541, 9.931948859054372747, 17.99999999999999645 ) ) ;
#18955=CARTESIAN_POINT ( 'NONE',  ( 56.68518183416157541, 10.06805114094562548, 11.99999999999999645 ) ) ;
#18974=CARTESIAN_POINT ( 'NONE',  ( 56.75231816583843170, 7.926799079670502124, 17.16943976678978245 ) ) ;
#18989=CARTESIAN_POINT ( 'NONE',  ( 52.78125000000000000, 8.343145750507600766, 11.00000000000000355 ) ) ;
#18998=CARTESIAN_POINT ( 'NONE',  ( 57.65625000000002132, 6.000000000000004441, 16.65685424949239390 ) ) ;
#19065=CARTESIAN_POINT ( 'NONE',  ( 58.27893183416158962, 8.825410453826341595, 11.97181229448535511 ) ) ;
#19076=CARTESIAN_POINT ( 'NONE',  ( 55.65393183416158251, 6.971812294485357775, 16.17458954617365663 ) ) ;
#19099=CARTESIAN_POINT ( 'NONE',  ( 53.65856816583844591, 7.028187705514647554, 16.31069182806492179 ) ) ;
#19109=SHAPE_REPRESENTATION_RELATIONSHIP ( 'NONE' , 'NONE' ,  #10226, #23619 ) ;
#19116=CARTESIAN_POINT ( 'NONE',  ( 51.00000000000000711, 12.82842712474617741, 12.17157287525379239 ) ) ;
#19127=CARTESIAN_POINT ( 'NONE',  ( 58.59375000000000711, 11.65685424949236193, 10.99999999999998401 ) ) ;
#19185=CARTESIAN_POINT ( 'NONE',  ( 53.77893183416158251, 8.825410453826341595, 11.97181229448535511 ) ) ;
#19196=CARTESIAN_POINT ( 'NONE',  ( 52.18518183416157541, 10.06805114094562548, 11.99999999999999645 ) ) ;
#19205=CARTESIAN_POINT ( 'NONE',  ( 56.75231816583843170, 7.926799079670502124, 17.16943976678978245 ) ) ;
#19214=CARTESIAN_POINT ( 'NONE',  ( 55.90856816583843880, 12.97181229448534978, 13.68930817193506755 ) ) ;
#19237=CARTESIAN_POINT ( 'NONE',  ( 53.90625000000000000, 13.99999999999999289, 13.34314575050759544 ) ) ;
#19292=CARTESIAN_POINT ( 'NONE',  ( 59.59143183416158962, 11.72490539043799984, 11.02818770551463246 ) ) ;
#19302=CARTESIAN_POINT ( 'NONE',  ( 55.27893183416158251, 8.825410453826341595, 11.97181229448535511 ) ) ;
#19313=CARTESIAN_POINT ( 'NONE',  ( 58.06481816583843170, 6.999999999999998224, 15.06805114094563436 ) ) ;
#19321=CARTESIAN_POINT ( 'NONE',  ( 57.84375000000000711, 8.757359312880723223, 18.00000000000000355 ) ) ;
#19325=CARTESIAN_POINT ( 'NONE',  ( 57.84375000000000711, 8.757359312880723223, 18.00000000000000355 ) ) ;
#19351=CARTESIAN_POINT ( 'NONE',  ( 56.71875000000000711, 14.00000000000000888, 16.65685424949235482 ) ) ;
#19405=CARTESIAN_POINT ( 'NONE',  ( 59.99999999999996447, 10.90022099756737717, 18.35387496708138499 ) ) ;
#19417=CARTESIAN_POINT ( 'NONE',  ( 59.96643183416158251, 6.028187705514633343, 13.27509460956200016 ) ) ;
#19428=CARTESIAN_POINT ( 'NONE',  ( 55.62731816583843170, 12.16943976678978601, 17.07320092032949432 ) ) ;
#19442=CARTESIAN_POINT ( 'NONE',  ( 50.09606816583843880, 11.17458954617364242, 11.97181229448534800 ) ) ;
#19455=( LENGTH_UNIT ( ) NAMED_UNIT ( * ) SI_UNIT ( .MILLI., .METRE. ) );
#19474=CARTESIAN_POINT ( 'NONE',  ( 57.12731816583843170, 12.87654654797634102, 17.78030770151602979 ) ) ;
#19489=CARTESIAN_POINT ( 'NONE',  ( 59.90625000000000711, 13.99999999999999289, 13.34314575050759544 ) ) ;
#19493=CARTESIAN_POINT ( 'NONE',  ( 58.34606816583844591, 8.411196891453267099, 19.02818770551464667 ) ) ;
#19494=MECHANICAL_DESIGN_GEOMETRIC_PRESENTATION_REPRESENTATION('',(#2279),#19869);
#19512=CARTESIAN_POINT ( 'NONE',  ( 56.90625000000000711, 12.99999999999999645, 13.75735931288070191 ) ) ;
#19531=CARTESIAN_POINT ( 'NONE',  ( 60.00000000000000711, 12.82842712474617741, 12.17157287525379239 ) ) ;
#19542=CARTESIAN_POINT ( 'NONE',  ( 59.77893183416158962, 8.411196891453236901, 10.97181229448535511 ) ) ;
#19551=CARTESIAN_POINT ( 'NONE',  ( 55.25231816583843170, 7.926799079670502124, 17.16943976678978245 ) ) ;
#19558=CARTESIAN_POINT ( 'NONE',  ( 57.65625000000002132, 7.000000000000003553, 16.24264068711929099 ) ) ;
#19560=CARTESIAN_POINT ( 'NONE',  ( 57.09375000000000711, 11.24264068711927322, 11.99999999999998934 ) ) ;
#19568=CARTESIAN_POINT ( 'NONE',  ( 57.84375000000000711, 8.757359312880723223, 18.00000000000000355 ) ) ;
#19587=CARTESIAN_POINT ( 'NONE',  ( 51.00000000000000711, 12.82842712474617741, 12.17157287525379239 ) ) ;
#19604=CARTESIAN_POINT ( 'NONE',  ( 57.78356816583844591, 8.275094609561968184, 11.02818770551464667 ) ) ;
#19622=CARTESIAN_POINT ( 'NONE',  ( 55.78125000000000711, 8.757359312880703683, 11.99999999999999822 ) ) ;
#19645=CARTESIAN_POINT ( 'NONE',  ( 59.99999999999729994, 11.15626659836185119, 18.14511749203898106 ) ) ;
#19654=CARTESIAN_POINT ( 'NONE',  ( 54.24768183416157541, 7.830560233210222876, 17.07320092032950498 ) ) ;
#19664=CARTESIAN_POINT ( 'NONE',  ( 53.84606816583843880, 8.825410453826357582, 18.02818770551464667 ) ) ;
#19671=CARTESIAN_POINT ( 'NONE',  ( 56.15625000000002132, 7.000000000000003553, 16.24264068711929099 ) ) ;
#19673=CARTESIAN_POINT ( 'NONE',  ( 58.59375000000000711, 11.24264068711927322, 11.99999999999998934 ) ) ;
#19682=CARTESIAN_POINT ( 'NONE',  ( 59.81250000000000711, 13.00000000000000000, 14.99999999999998757 ) ) ;
#19701=CARTESIAN_POINT ( 'NONE',  ( 58.81481816583843170, 14.00000000000000178, 14.93194885905434610 ) ) ;
#19724=CARTESIAN_POINT ( 'NONE',  ( 54.56250000000000711, 5.999999999999996447, 15.00000000000001599 ) ) ;
#19731=CARTESIAN_POINT ( 'NONE',  ( 60.52893183416158251, 11.58880310854676132, 19.02818770551463956 ) ) ;
#19742=CARTESIAN_POINT ( 'NONE',  ( 57.56250000000000000, 6.999999999999997335, 15.00000000000000533 ) ) ;
#19762=CARTESIAN_POINT ( 'NONE',  ( 60.00000000000001421, 13.04648002170960197, 12.38962577221721340 ) ) ;
#19774=CARTESIAN_POINT ( 'NONE',  ( 54.62268183416157541, 12.78030770151606177, 17.87654654797631792 ) ) ;
#19777=( BOUNDED_SURFACE ( )  B_SPLINE_SURFACE ( 3, 2, ( 
 ( #10273, #15999, #19682, #17447, #21353, #8474, #19805, #13975, #1241, #1482, #8824, #12182, #10398, #17788, #3287, #5083, #8579, #15885, #7011, #6772, #14088, #6894, #10629, #19568, #21588, #3162, #1360, #14214, #5202, #12542, #16697, #18483, #7379, #7488, #5554, #14931, #19925, #159, #9406, #14806, #16467, #273, #9056, #23644, #5673, #5324, #18246, #7608, #1601, #11088, #22184, #20386, #12667, #18135, #16347, #5798, #13126, #14447, #10970, #3631, #14687, #12776, #8941, #20028, #20142, #2066, #10752, #18025, #21839, #1713, #21944, #3747, #16233, #23519, #18372, #3875, #7133, #21712, #7257, #3525, #10858, #14573, #1953, #5440, #12886, #9291, #1831, #9182, #22055, #20271, #46, #16580, #13006, #11209, #22552, #13710, #13591 ),
 ( #2427, #17176, #20857, #6159, #8091, #18604, #4349, #11574, #9758, #6274, #10011, #11806, #630, #758, #13482, #8199, #13241, #15400, #2668, #22664, #17056, #17299, #2317, #16940, #4464, #22302, #18842, #864, #2189, #11686, #15512, #3992, #5915, #11452, #9650, #22780, #6389, #7732, #4237, #20629, #7960, #6035, #9527, #15280, #20743, #11332, #18955, #16825, #2540, #18727, #403, #15044, #13361, #20508, #4113, #9884, #517, #19076, #7839, #15160, #22421, #19302, #23023, #23249, #8668, #8551, #3013, #2893, #15753, #1328, #21320, #21204, #19654, #1449, #8786, #17532, #6858, #10241, #8310, #15858, #5056, #4818, #6745, #14052, #20971, #15633, #15966, #23378, #12276, #4592, #6981, #10365, #4706, #11927, #19196, #6628, #22902 ),
 ( #23132, #3137, #6518, #1097, #8443, #13948, #14183, #21443, #4940, #17654, #12150, #19417, #12389, #19542, #1214, #3255, #16091, #2780, #10479, #10602, #17760, #13837, #17876, #10120, #17413, #982, #21092, #12039, #8910, #1927, #16670, #5526, #21560, #14659, #9379, #21, #9153, #22029, #3719, #12860, #14777, #16556, #12980, #3378, #5646, #10718, #12638, #20116, #132, #16325, #10944, #1572, #11061, #9269, #244, #18223, #16205, #14299, #5173, #14546, #20244, #3851, #12514, #19897, #7354, #7461, #11186, #5295, #19774, #18460, #17995, #12751, #18347, #2041, #16439, #23491, #7104, #21916, #21812, #20003, #14421, #21684, #3499, #1806, #10834, #18108, #1688, #9032, #23616, #7230, #5414, #3605, #18932, #15022, #22276, #15251, #11301 ),
 ( #11549, #2518, #15374, #18575, #16792, #5889, #9852, #17149, #3965, #2287, #18697, #15134, #4084, #14898, #493, #16916, #11664, #6007, #22518, #727, #8060, #7705, #4208, #2156, #13332, #18818, #5774, #13101, #605, #7579, #372, #22155, #20357, #9493, #13213, #7931, #20482, #6128, #11422, #9625, #7816, #22397, #20600, #2403, #9735, #17030, #13457, #20719, #4323, #3202, #21633, #18061, #17825, #12457, #3091, #14369, #10787, #1757, #19724, #17714, #18174, #6691, #16040, #16274, #23566, #14009, #14130, #8862, #1641, #3449, #6809, #15811, #21752, #23083, #14254, #5238, #8986, #10666, #19842, #21267, #16159, #23328, #21511, #7173, #5363, #14489, #3321, #12582, #17942, #19959, #1277, #12707, #3559, #10896, #5122, #4887, #21396 ),
 ( #10549, #12225, #1523, #6939, #8614, #23446, #7051, #19493, #10433, #15918, #23196, #5014, #12343, #19604, #1391, #8732, #5832, #9094, #18643, #14843, #18288, #7414, #16387, #79, #440, #11243, #5953, #22221, #16617, #18409, #5715, #1872, #15084, #9220, #22097, #9572, #14609, #7764, #1986, #20185, #18517, #3792, #7301, #196, #9441, #22339, #11132, #14970, #11366, #9325, #13047, #20069, #7651, #4031, #18770, #20306, #11007, #11497, #23685, #7526, #16865, #13278, #21870, #14723, #2103, #2228, #20421, #21981, #5476, #20547, #12811, #3907, #13160, #4151, #16735, #3671, #16503, #317, #5598, #12924, #4952, #8677, #10490, #23032, #23143, #21214, #6872, #11940, #15869, #1341, #6754, #8454, #15977, #993, #15641, #21332, #20983 ),
 ( #3024, #23262, #12400, #4604, #10133, #8318, #14195, #21453, #6400, #2904, #19313, #6642, #4716, #17308, #15761, #1107, #5066, #13956, #2682, #4828, #17426, #875, #8209, #12047, #19205, #10021, #17539, #22792, #12160, #8561, #2791, #6527, #22913, #10250, #12287, #14066, #19428, #10375, #13846, #21101, #19551, #17662, #1223, #15526, #13720, #3146, #17770, #21926, #8922, #6990, #7238, #3729, #3508, #5422, #12759, #19664, #14310, #7361, #22037, #10953, #3267, #20013, #14790, #3613, #14556, #11070, #9162, #18230, #20123, #5535, #18355, #5305, #1936, #9277, #10843, #1814, #16450, #10613, #21569, #14667, #5654, #31, #17884, #12870, #1459, #16562, #21821, #140, #7469, #8802, #16104, #23388, #5182, #12647, #12524, #19786, #7115 ),
 ( #16331, #3386, #10730, #18007, #1583, #23625, #16215, #23500, #14430, #19906, #21695, #18119, #1695, #9039, #6015, #7941, #616, #3975, #15385, #18940, #20253, #11434, #2411, #6141, #7824, #17038, #3859, #13342, #20491, #18708, #15261, #2525, #20727, #9634, #9744, #15143, #17159, #22164, #22530, #11671, #13467, #2297, #9862, #11309, #2166, #4331, #9505, #18826, #738, #16924, #13223, #5781, #501, #22407, #11557, #8070, #11194, #22649, #253, #18585, #7588, #12988, #22283, #18469, #2047, #9387, #20609, #13109, #16802, #16681, #382, #14906, #4219, #20367, #7714, #4092, #5900, #15029, #15495, #12257, #6376, #12018, #6724, #11785, #21299, #15615, #17395, #15735, #962, #4450, #13818, #6613, #1198, #10462, #1310, #4574, #23007 ) ),
 .UNSPECIFIED., .T., .F., .F. ) 
 B_SPLINE_SURFACE_WITH_KNOTS ( ( 4, 3, 4 ),
 ( 3, 2, 2, 2, 2, 2, 2, 2, 2, 2, 2, 2, 2, 2, 2, 2, 2, 2, 2, 2, 2, 2, 2, 2, 2, 2, 2, 2, 2, 2, 2, 2, 2, 2, 2, 2, 2, 2, 2, 2, 2, 2, 2, 2, 2, 2, 2, 2, 3 ),
 ( 0.000000000000000000, 0.5000000000000000000, 1.000000000000000000 ),
 ( 0.000000000000000000, 0.02083333333333333218, 0.04166666666666666435, 0.06250000000000000000, 0.08333333333333332871, 0.1041666666666666713, 0.1250000000000000000, 0.1458333333333333426, 0.1666666666666666574, 0.1875000000000000000, 0.2083333333333333426, 0.2291666666666666574, 0.2500000000000000000, 0.2708333333333333148, 0.2916666666666666852, 0.3125000000000000000, 0.3333333333333333148, 0.3541666666666666852, 0.3750000000000000000, 0.3958333333333333148, 0.4166666666666666852, 0.4375000000000000000, 0.4583333333333333148, 0.4791666666666666852, 0.5000000000000000000, 0.5208333333333333703, 0.5416666666666666297, 0.5625000000000000000, 0.5833333333333333703, 0.6041666666666666297, 0.6250000000000000000, 0.6458333333333333703, 0.6666666666666666297, 0.6875000000000000000, 0.7083333333333333703, 0.7291666666666666297, 0.7500000000000000000, 0.7708333333333333703, 0.7916666666666666297, 0.8125000000000000000, 0.8333333333333333703, 0.8541666666666666297, 0.8750000000000000000, 0.8958333333333333703, 0.9166666666666666297, 0.9375000000000000000, 0.9583333333333333703, 0.9791666666666666297, 1.000000000000000000 ),
 .UNSPECIFIED. ) 
 GEOMETRIC_REPRESENTATION_ITEM ( )  RATIONAL_B_SPLINE_SURFACE ( (
 ( 1.000000000000000000, 0.9238795325112867385, 1.000000000000000000, 0.9238795325112867385, 1.000000000000000000, 0.9238795325112867385, 1.000000000000000000, 0.9238795325112867385, 1.000000000000000000, 0.9238795325112867385, 1.000000000000000000, 0.9238795325112867385, 1.000000000000000000, 0.9238795325112867385, 1.000000000000000000, 0.9238795325112867385, 1.000000000000000000, 0.9238795325112867385, 1.000000000000000000, 0.9238795325112867385, 1.000000000000000000, 0.9238795325112867385, 1.000000000000000000, 0.9238795325112867385, 1.000000000000000000, 0.9238795325112867385, 1.000000000000000000, 0.9238795325112867385, 1.000000000000000000, 0.9238795325112867385, 1.000000000000000000, 0.9238795325112867385, 1.000000000000000000, 0.9238795325112867385, 1.000000000000000000, 0.9238795325112867385, 1.000000000000000000, 0.9238795325112867385, 1.000000000000000000, 0.9238795325112867385, 1.000000000000000000, 0.9238795325112867385, 1.000000000000000000, 0.9238795325112867385, 1.000000000000000000, 0.9238795325112867385, 1.000000000000000000, 0.9238795325112867385, 1.000000000000000000, 0.9238795325112867385, 1.000000000000000000, 0.9238795325112867385, 1.000000000000000000, 0.9238795325112867385, 1.000000000000000000, 0.9238795325112867385, 1.000000000000000000, 0.9238795325112867385, 1.000000000000000000, 0.9238795325112867385, 1.000000000000000000, 0.9238795325112867385, 1.000000000000000000, 0.9238795325112867385, 1.000000000000000000, 0.9238795325112867385, 1.000000000000000000, 0.9238795325112867385, 1.000000000000000000, 0.9238795325112867385, 1.000000000000000000, 0.9238795325112867385, 1.000000000000000000, 0.9238795325112867385, 1.000000000000000000, 0.9238795325112867385, 1.000000000000000000, 0.9238795325112867385, 1.000000000000000000, 0.9238795325112867385, 1.000000000000000000, 0.9238795325112867385, 1.000000000000000000, 0.9238795325112867385, 1.000000000000000000, 0.9238795325112867385, 1.000000000000000000, 0.9238795325112867385, 1.000000000000000000, 0.9238795325112867385, 1.000000000000000000, 0.9238795325112867385, 1.000000000000000000, 0.9238795325112867385, 1.000000000000000000, 0.9238795325112867385, 1.000000000000000000),
 ( 0.3333333333333333703, 0.3079598441704289313, 0.3333333333333333703, 0.3079598441704289313, 0.3333333333333333703, 0.3079598441704289313, 0.3333333333333333703, 0.3079598441704289313, 0.3333333333333333703, 0.3079598441704289313, 0.3333333333333333703, 0.3079598441704289313, 0.3333333333333333703, 0.3079598441704289313, 0.3333333333333333703, 0.3079598441704289313, 0.3333333333333333703, 0.3079598441704289313, 0.3333333333333333703, 0.3079598441704289313, 0.3333333333333333703, 0.3079598441704289313, 0.3333333333333333703, 0.3079598441704289313, 0.3333333333333333703, 0.3079598441704289313, 0.3333333333333333703, 0.3079598441704289313, 0.3333333333333333703, 0.3079598441704289313, 0.3333333333333333703, 0.3079598441704289313, 0.3333333333333333703, 0.3079598441704289313, 0.3333333333333333703, 0.3079598441704289313, 0.3333333333333333703, 0.3079598441704289313, 0.3333333333333333703, 0.3079598441704289313, 0.3333333333333333703, 0.3079598441704289313, 0.3333333333333333703, 0.3079598441704289313, 0.3333333333333333703, 0.3079598441704289313, 0.3333333333333333703, 0.3079598441704289313, 0.3333333333333333703, 0.3079598441704289313, 0.3333333333333333703, 0.3079598441704289313, 0.3333333333333333703, 0.3079598441704289313, 0.3333333333333333703, 0.3079598441704289313, 0.3333333333333333703, 0.3079598441704289313, 0.3333333333333333703, 0.3079598441704289313, 0.3333333333333333703, 0.3079598441704289313, 0.3333333333333333703, 0.3079598441704289313, 0.3333333333333333703, 0.3079598441704289313, 0.3333333333333333703, 0.3079598441704289313, 0.3333333333333333703, 0.3079598441704289313, 0.3333333333333333703, 0.3079598441704289313, 0.3333333333333333703, 0.3079598441704289313, 0.3333333333333333703, 0.3079598441704289313, 0.3333333333333333703, 0.3079598441704289313, 0.3333333333333333703, 0.3079598441704289313, 0.3333333333333333703, 0.3079598441704289313, 0.3333333333333333703, 0.3079598441704289313, 0.3333333333333333703, 0.3079598441704289313, 0.3333333333333333703, 0.3079598441704289313, 0.3333333333333333703, 0.3079598441704289313, 0.3333333333333333703, 0.3079598441704289313, 0.3333333333333333703, 0.3079598441704289313, 0.3333333333333333703, 0.3079598441704289313, 0.3333333333333333703),
 ( 0.3333333333333333703, 0.3079598441704289313, 0.3333333333333333703, 0.3079598441704289313, 0.3333333333333333703, 0.3079598441704289313, 0.3333333333333333703, 0.3079598441704289313, 0.3333333333333333703, 0.3079598441704289313, 0.3333333333333333703, 0.3079598441704289313, 0.3333333333333333703, 0.3079598441704289313, 0.3333333333333333703, 0.3079598441704289313, 0.3333333333333333703, 0.3079598441704289313, 0.3333333333333333703, 0.3079598441704289313, 0.3333333333333333703, 0.3079598441704289313, 0.3333333333333333703, 0.3079598441704289313, 0.3333333333333333703, 0.3079598441704289313, 0.3333333333333333703, 0.3079598441704289313, 0.3333333333333333703, 0.3079598441704289313, 0.3333333333333333703, 0.3079598441704289313, 0.3333333333333333703, 0.3079598441704289313, 0.3333333333333333703, 0.3079598441704289313, 0.3333333333333333703, 0.3079598441704289313, 0.3333333333333333703, 0.3079598441704289313, 0.3333333333333333703, 0.3079598441704289313, 0.3333333333333333703, 0.3079598441704289313, 0.3333333333333333703, 0.3079598441704289313, 0.3333333333333333703, 0.3079598441704289313, 0.3333333333333333703, 0.3079598441704289313, 0.3333333333333333703, 0.3079598441704289313, 0.3333333333333333703, 0.3079598441704289313, 0.3333333333333333703, 0.3079598441704289313, 0.3333333333333333703, 0.3079598441704289313, 0.3333333333333333703, 0.3079598441704289313, 0.3333333333333333703, 0.3079598441704289313, 0.3333333333333333703, 0.3079598441704289313, 0.3333333333333333703, 0.3079598441704289313, 0.3333333333333333703, 0.3079598441704289313, 0.3333333333333333703, 0.3079598441704289313, 0.3333333333333333703, 0.3079598441704289313, 0.3333333333333333703, 0.3079598441704289313, 0.3333333333333333703, 0.3079598441704289313, 0.3333333333333333703, 0.3079598441704289313, 0.3333333333333333703, 0.3079598441704289313, 0.3333333333333333703, 0.3079598441704289313, 0.3333333333333333703, 0.3079598441704289313, 0.3333333333333333703, 0.3079598441704289313, 0.3333333333333333703, 0.3079598441704289313, 0.3333333333333333703, 0.3079598441704289313, 0.3333333333333333703, 0.3079598441704289313, 0.3333333333333333703, 0.3079598441704289313, 0.3333333333333333703, 0.3079598441704289313, 0.3333333333333333703),
 ( 1.000000000000000000, 0.9238795325112867385, 1.000000000000000000, 0.9238795325112867385, 1.000000000000000000, 0.9238795325112867385, 1.000000000000000000, 0.9238795325112867385, 1.000000000000000000, 0.9238795325112867385, 1.000000000000000000, 0.9238795325112867385, 1.000000000000000000, 0.9238795325112867385, 1.000000000000000000, 0.9238795325112867385, 1.000000000000000000, 0.9238795325112867385, 1.000000000000000000, 0.9238795325112867385, 1.000000000000000000, 0.9238795325112867385, 1.000000000000000000, 0.9238795325112867385, 1.000000000000000000, 0.9238795325112867385, 1.000000000000000000, 0.9238795325112867385, 1.000000000000000000, 0.9238795325112867385, 1.000000000000000000, 0.9238795325112867385, 1.000000000000000000, 0.9238795325112867385, 1.000000000000000000, 0.9238795325112867385, 1.000000000000000000, 0.9238795325112867385, 1.000000000000000000, 0.9238795325112867385, 1.000000000000000000, 0.9238795325112867385, 1.000000000000000000, 0.9238795325112867385, 1.000000000000000000, 0.9238795325112867385, 1.000000000000000000, 0.9238795325112867385, 1.000000000000000000, 0.9238795325112867385, 1.000000000000000000, 0.9238795325112867385, 1.000000000000000000, 0.9238795325112867385, 1.000000000000000000, 0.9238795325112867385, 1.000000000000000000, 0.9238795325112867385, 1.000000000000000000, 0.9238795325112867385, 1.000000000000000000, 0.9238795325112867385, 1.000000000000000000, 0.9238795325112867385, 1.000000000000000000, 0.9238795325112867385, 1.000000000000000000, 0.9238795325112867385, 1.000000000000000000, 0.9238795325112867385, 1.000000000000000000, 0.9238795325112867385, 1.000000000000000000, 0.9238795325112867385, 1.000000000000000000, 0.9238795325112867385, 1.000000000000000000, 0.9238795325112867385, 1.000000000000000000, 0.9238795325112867385, 1.000000000000000000, 0.9238795325112867385, 1.000000000000000000, 0.9238795325112867385, 1.000000000000000000, 0.9238795325112867385, 1.000000000000000000, 0.9238795325112867385, 1.000000000000000000, 0.9238795325112867385, 1.000000000000000000, 0.9238795325112867385, 1.000000000000000000, 0.9238795325112867385, 1.000000000000000000, 0.9238795325112867385, 1.000000000000000000),
 ( 0.3333333333333333703, 0.3079598441704289313, 0.3333333333333333703, 0.3079598441704289313, 0.3333333333333333703, 0.3079598441704289313, 0.3333333333333333703, 0.3079598441704289313, 0.3333333333333333703, 0.3079598441704289313, 0.3333333333333333703, 0.3079598441704289313, 0.3333333333333333703, 0.3079598441704289313, 0.3333333333333333703, 0.3079598441704289313, 0.3333333333333333703, 0.3079598441704289313, 0.3333333333333333703, 0.3079598441704289313, 0.3333333333333333703, 0.3079598441704289313, 0.3333333333333333703, 0.3079598441704289313, 0.3333333333333333703, 0.3079598441704289313, 0.3333333333333333703, 0.3079598441704289313, 0.3333333333333333703, 0.3079598441704289313, 0.3333333333333333703, 0.3079598441704289313, 0.3333333333333333703, 0.3079598441704289313, 0.3333333333333333703, 0.3079598441704289313, 0.3333333333333333703, 0.3079598441704289313, 0.3333333333333333703, 0.3079598441704289313, 0.3333333333333333703, 0.3079598441704289313, 0.3333333333333333703, 0.3079598441704289313, 0.3333333333333333703, 0.3079598441704289313, 0.3333333333333333703, 0.3079598441704289313, 0.3333333333333333703, 0.3079598441704289313, 0.3333333333333333703, 0.3079598441704289313, 0.3333333333333333703, 0.3079598441704289313, 0.3333333333333333703, 0.3079598441704289313, 0.3333333333333333703, 0.3079598441704289313, 0.3333333333333333703, 0.3079598441704289313, 0.3333333333333333703, 0.3079598441704289313, 0.3333333333333333703, 0.3079598441704289313, 0.3333333333333333703, 0.3079598441704289313, 0.3333333333333333703, 0.3079598441704289313, 0.3333333333333333703, 0.3079598441704289313, 0.3333333333333333703, 0.3079598441704289313, 0.3333333333333333703, 0.3079598441704289313, 0.3333333333333333703, 0.3079598441704289313, 0.3333333333333333703, 0.3079598441704289313, 0.3333333333333333703, 0.3079598441704289313, 0.3333333333333333703, 0.3079598441704289313, 0.3333333333333333703, 0.3079598441704289313, 0.3333333333333333703, 0.3079598441704289313, 0.3333333333333333703, 0.3079598441704289313, 0.3333333333333333703, 0.3079598441704289313, 0.3333333333333333703, 0.3079598441704289313, 0.3333333333333333703, 0.3079598441704289313, 0.3333333333333333703, 0.3079598441704289313, 0.3333333333333333703),
 ( 0.3333333333333333703, 0.3079598441704289313, 0.3333333333333333703, 0.3079598441704289313, 0.3333333333333333703, 0.3079598441704289313, 0.3333333333333333703, 0.3079598441704289313, 0.3333333333333333703, 0.3079598441704289313, 0.3333333333333333703, 0.3079598441704289313, 0.3333333333333333703, 0.3079598441704289313, 0.3333333333333333703, 0.3079598441704289313, 0.3333333333333333703, 0.3079598441704289313, 0.3333333333333333703, 0.3079598441704289313, 0.3333333333333333703, 0.3079598441704289313, 0.3333333333333333703, 0.3079598441704289313, 0.3333333333333333703, 0.3079598441704289313, 0.3333333333333333703, 0.3079598441704289313, 0.3333333333333333703, 0.3079598441704289313, 0.3333333333333333703, 0.3079598441704289313, 0.3333333333333333703, 0.3079598441704289313, 0.3333333333333333703, 0.3079598441704289313, 0.3333333333333333703, 0.3079598441704289313, 0.3333333333333333703, 0.3079598441704289313, 0.3333333333333333703, 0.3079598441704289313, 0.3333333333333333703, 0.3079598441704289313, 0.3333333333333333703, 0.3079598441704289313, 0.3333333333333333703, 0.3079598441704289313, 0.3333333333333333703, 0.3079598441704289313, 0.3333333333333333703, 0.3079598441704289313, 0.3333333333333333703, 0.3079598441704289313, 0.3333333333333333703, 0.3079598441704289313, 0.3333333333333333703, 0.3079598441704289313, 0.3333333333333333703, 0.3079598441704289313, 0.3333333333333333703, 0.3079598441704289313, 0.3333333333333333703, 0.3079598441704289313, 0.3333333333333333703, 0.3079598441704289313, 0.3333333333333333703, 0.3079598441704289313, 0.3333333333333333703, 0.3079598441704289313, 0.3333333333333333703, 0.3079598441704289313, 0.3333333333333333703, 0.3079598441704289313, 0.3333333333333333703, 0.3079598441704289313, 0.3333333333333333703, 0.3079598441704289313, 0.3333333333333333703, 0.3079598441704289313, 0.3333333333333333703, 0.3079598441704289313, 0.3333333333333333703, 0.3079598441704289313, 0.3333333333333333703, 0.3079598441704289313, 0.3333333333333333703, 0.3079598441704289313, 0.3333333333333333703, 0.3079598441704289313, 0.3333333333333333703, 0.3079598441704289313, 0.3333333333333333703, 0.3079598441704289313, 0.3333333333333333703, 0.3079598441704289313, 0.3333333333333333703),
 ( 1.000000000000000000, 0.9238795325112867385, 1.000000000000000000, 0.9238795325112867385, 1.000000000000000000, 0.9238795325112867385, 1.000000000000000000, 0.9238795325112867385, 1.000000000000000000, 0.9238795325112867385, 1.000000000000000000, 0.9238795325112867385, 1.000000000000000000, 0.9238795325112867385, 1.000000000000000000, 0.9238795325112867385, 1.000000000000000000, 0.9238795325112867385, 1.000000000000000000, 0.9238795325112867385, 1.000000000000000000, 0.9238795325112867385, 1.000000000000000000, 0.9238795325112867385, 1.000000000000000000, 0.9238795325112867385, 1.000000000000000000, 0.9238795325112867385, 1.000000000000000000, 0.9238795325112867385, 1.000000000000000000, 0.9238795325112867385, 1.000000000000000000, 0.9238795325112867385, 1.000000000000000000, 0.9238795325112867385, 1.000000000000000000, 0.9238795325112867385, 1.000000000000000000, 0.9238795325112867385, 1.000000000000000000, 0.9238795325112867385, 1.000000000000000000, 0.9238795325112867385, 1.000000000000000000, 0.9238795325112867385, 1.000000000000000000, 0.9238795325112867385, 1.000000000000000000, 0.9238795325112867385, 1.000000000000000000, 0.9238795325112867385, 1.000000000000000000, 0.9238795325112867385, 1.000000000000000000, 0.9238795325112867385, 1.000000000000000000, 0.9238795325112867385, 1.000000000000000000, 0.9238795325112867385, 1.000000000000000000, 0.9238795325112867385, 1.000000000000000000, 0.9238795325112867385, 1.000000000000000000, 0.9238795325112867385, 1.000000000000000000, 0.9238795325112867385, 1.000000000000000000, 0.9238795325112867385, 1.000000000000000000, 0.9238795325112867385, 1.000000000000000000, 0.9238795325112867385, 1.000000000000000000, 0.9238795325112867385, 1.000000000000000000, 0.9238795325112867385, 1.000000000000000000, 0.9238795325112867385, 1.000000000000000000, 0.9238795325112867385, 1.000000000000000000, 0.9238795325112867385, 1.000000000000000000, 0.9238795325112867385, 1.000000000000000000, 0.9238795325112867385, 1.000000000000000000, 0.9238795325112867385, 1.000000000000000000, 0.9238795325112867385, 1.000000000000000000, 0.9238795325112867385, 1.000000000000000000, 0.9238795325112867385, 1.000000000000000000) ) ) 
 REPRESENTATION_ITEM ( '' )  SURFACE ( )  );
#19786=CARTESIAN_POINT ( 'NONE',  ( 50.09606816583843880, 11.17458954617364242, 11.97181229448534800 ) ) ;
#19797=CARTESIAN_POINT ( 'NONE',  ( 51.03356816583844591, 11.31069182806492712, 17.97181229448534623 ) ) ;
#19805=CARTESIAN_POINT ( 'NONE',  ( 59.43750000000000711, 10.00000000000000711, 17.99999999999999645 ) ) ;
#19823=CARTESIAN_POINT ( 'NONE',  ( 57.50231816583843170, 12.78030770151603868, 12.12345345202365188 ) ) ;
#19837=CARTESIAN_POINT ( 'NONE',  ( 60.00000000000000711, 12.82842712474617741, 12.17157287525379239 ) ) ;
#19842=CARTESIAN_POINT ( 'NONE',  ( 52.68750000000000711, 9.999999999999978684, 10.99999999999999645 ) ) ;
#19853=CARTESIAN_POINT ( 'NONE',  ( 57.90393183416158251, 14.02818770551463956, 13.41119689145323335 ) ) ;
#19863=CARTESIAN_POINT ( 'NONE',  ( 54.84375000000000711, 8.757359312880723223, 18.00000000000000711 ) ) ;
#19869=( GEOMETRIC_REPRESENTATION_CONTEXT ( 3 ) GLOBAL_UNCERTAINTY_ASSIGNED_CONTEXT ( ( #17221 ) ) GLOBAL_UNIT_ASSIGNED_CONTEXT ( ( #19944, #18624, #11477 ) ) REPRESENTATION_CONTEXT ( 'NONE', 'WORKASPACE' ) );
#19887=CARTESIAN_POINT ( 'NONE',  ( 59.99999999999997868, 10.93287452463206577, 18.30488221186498521 ) ) ;
#19897=CARTESIAN_POINT ( 'NONE',  ( 55.09143183416158962, 11.72490539043799984, 11.02818770551463246 ) ) ;
#19906=CARTESIAN_POINT ( 'NONE',  ( 59.15625000000002132, 7.000000000000003553, 16.24264068711929099 ) ) ;
#19913=CARTESIAN_POINT ( 'NONE',  ( 54.56250000000000711, 6.999999999999997335, 15.00000000000000533 ) ) ;
#19917=CARTESIAN_POINT ( 'NONE',  ( 52.50000000000000711, 12.12132034355963484, 12.87867965644034740 ) ) ;
#19925=CARTESIAN_POINT ( 'NONE',  ( 56.62500000000000000, 12.12132034355964727, 17.12132034355963484 ) ) ;
#19942=CARTESIAN_POINT ( 'NONE',  ( 56.00231816583843170, 12.78030770151603868, 12.12345345202365188 ) ) ;
#19944=( LENGTH_UNIT ( ) NAMED_UNIT ( * ) SI_UNIT ( .MILLI., .METRE. ) );
#19955=CARTESIAN_POINT ( 'NONE',  ( 56.15625000000001421, 6.000000000000004441, 16.65685424949239390 ) ) ;
#19959=CARTESIAN_POINT ( 'NONE',  ( 51.65625000000000711, 6.000000000000004441, 16.65685424949239390 ) ) ;
#19967=CARTESIAN_POINT ( 'NONE',  ( 59.31018183416157541, 14.00000000000000000, 15.06805114094561304 ) ) ;
#19974=CARTESIAN_POINT ( 'NONE',  ( 58.96875000000000711, 6.999999999999992006, 13.75735931288071967 ) ) ;
#20003=CARTESIAN_POINT ( 'NONE',  ( 53.59143183416158962, 11.72490539043799984, 11.02818770551463246 ) ) ;
#20013=CARTESIAN_POINT ( 'NONE',  ( 53.28356816583845301, 8.689308171935074654, 12.02818770551464489 ) ) ;
#20018=CARTESIAN_POINT ( 'NONE',  ( 55.59375000000000711, 11.24264068711927322, 11.99999999999998934 ) ) ;
#20020=CARTESIAN_POINT ( 'NONE',  ( 53.15625000000001421, 7.000000000000003553, 16.24264068711929099 ) ) ;
#20028=CARTESIAN_POINT ( 'NONE',  ( 54.09375000000000711, 11.24264068711927322, 11.99999999999998934 ) ) ;
#20047=CARTESIAN_POINT ( 'NONE',  ( 51.87731816583844591, 7.123453452023657206, 12.21969229848395599 ) ) ;
#20064=CARTESIAN_POINT ( 'NONE',  ( 57.93750000000000000, 10.00000000000001776, 18.99999999999999645 ) ) ;
#20069=CARTESIAN_POINT ( 'NONE',  ( 54.22106816583844591, 14.02818770551465377, 16.58880310854672757 ) ) ;
#20079=CARTESIAN_POINT ( 'NONE',  ( 56.40393183416158251, 14.02818770551463956, 13.41119689145323335 ) ) ;
#20087=CARTESIAN_POINT ( 'NONE',  ( 51.93750000000000711, 10.00000000000000711, 17.99999999999999645 ) ) ;
#20116=CARTESIAN_POINT ( 'NONE',  ( 56.59143183416158962, 11.72490539043799984, 11.02818770551463246 ) ) ;
#20123=CARTESIAN_POINT ( 'NONE',  ( 52.62731816583844591, 12.16943976678978601, 17.07320092032949432 ) ) ;
#20130=CARTESIAN_POINT ( 'NONE',  ( 51.56250000000000711, 6.999999999999997335, 15.00000000000000533 ) ) ;
#20132=CARTESIAN_POINT ( 'NONE',  ( 55.78125000000000000, 8.757359312880703683, 11.99999999999999822 ) ) ;
#20142=CARTESIAN_POINT ( 'NONE',  ( 54.00000000000000711, 12.12132034355963484, 12.87867965644034740 ) ) ;
#20163=CARTESIAN_POINT ( 'NONE',  ( 58.90856816583844591, 12.97181229448534978, 13.68930817193506755 ) ) ;
#20181=CARTESIAN_POINT ( 'NONE',  ( 53.25000000000000711, 7.171572875253819923, 17.82842712474619873 ) ) ;
#20185=CARTESIAN_POINT ( 'NONE',  ( 55.34606816583843880, 8.411196891453267099, 19.02818770551464667 ) ) ;
#20197=CARTESIAN_POINT ( 'NONE',  ( 56.68518183416157541, 10.06805114094561659, 10.99999999999999645 ) ) ;
#20206=CARTESIAN_POINT ( 'NONE',  ( 52.59375000000000711, 11.24264068711927322, 11.99999999999998934 ) ) ;
#20244=CARTESIAN_POINT ( 'NONE',  ( 55.37268183416157541, 7.219692298483935566, 12.12345345202367675 ) ) ;
#20253=CARTESIAN_POINT ( 'NONE',  ( 58.12500000000000000, 12.12132034355964727, 17.12132034355963484 ) ) ;
#20260=CARTESIAN_POINT ( 'NONE',  ( 60.15393183416158962, 6.971812294485357775, 16.17458954617365663 ) ) ;
#20263=CARTESIAN_POINT ( 'NONE',  ( 51.37500000000000711, 7.878679656440349177, 12.87867965644035984 ) ) ;
#20271=CARTESIAN_POINT ( 'NONE',  ( 51.65625000000000711, 7.000000000000003553, 16.24264068711929099 ) ) ;
#20288=CARTESIAN_POINT ( 'NONE',  ( 50.56481816583844591, 5.999999999999996447, 15.06805114094564502 ) ) ;
#20302=CARTESIAN_POINT ( 'NONE',  ( 58.78125000000000711, 8.343145750507600766, 11.00000000000000355 ) ) ;
#20306=CARTESIAN_POINT ( 'NONE',  ( 53.84606816583843880, 8.411196891453267099, 19.02818770551464667 ) ) ;
#20314=CARTESIAN_POINT ( 'NONE',  ( 56.87268183416158962, 7.219692298483935566, 12.12345345202367675 ) ) ;
#20357=CARTESIAN_POINT ( 'NONE',  ( 57.00000000000000000, 12.82842712474617741, 12.17157287525379239 ) ) ;
#20367=CARTESIAN_POINT ( 'NONE',  ( 53.15625000000001421, 7.000000000000003553, 16.24264068711929099 ) ) ;
#20375=CARTESIAN_POINT ( 'NONE',  ( 51.84375000000001421, 8.757359312880723223, 18.00000000000000355 ) ) ;
#20377=CARTESIAN_POINT ( 'NONE',  ( 54.09375000000000711, 11.24264068711927322, 11.99999999999998934 ) ) ;
#20386=CARTESIAN_POINT ( 'NONE',  ( 55.21875000000000000, 13.00000000000000711, 16.24264068711927322 ) ) ;
#20404=CARTESIAN_POINT ( 'NONE',  ( 50.09606816583843880, 11.58880310854672935, 10.97181229448534445 ) ) ;
#20417=CARTESIAN_POINT ( 'NONE',  ( 57.18750000000000000, 9.999999999999978684, 10.99999999999999645 ) ) ;
#20421=CARTESIAN_POINT ( 'NONE',  ( 52.81481816583844591, 14.00000000000000178, 14.93194885905434610 ) ) ;
#20434=CARTESIAN_POINT ( 'NONE',  ( 52.65393183416158251, 5.971812294485358663, 16.58880310854675599 ) ) ;
#20441=CARTESIAN_POINT ( 'NONE',  ( 52.96875000000000000, 6.999999999999992006, 13.75735931288071967 ) ) ;
#20482=CARTESIAN_POINT ( 'NONE',  ( 56.62500000000000000, 12.82842712474620228, 17.82842712474617386 ) ) ;
#20491=CARTESIAN_POINT ( 'NONE',  ( 57.37500000000000000, 7.878679656440349177, 12.87867965644035984 ) ) ;
#20497=CARTESIAN_POINT ( 'NONE',  ( 55.56018183416157541, 7.000000000000000000, 14.93194885905437097 ) ) ;
#20508=CARTESIAN_POINT ( 'NONE',  ( 56.02893183416158962, 11.17458954617365663, 18.02818770551464311 ) ) ;
#20524=CARTESIAN_POINT ( 'NONE',  ( 54.22106816583844591, 14.02818770551465377, 16.58880310854672757 ) ) ;
#20541=CARTESIAN_POINT ( 'NONE',  ( 52.59375000000000711, 11.65685424949236015, 10.99999999999998579 ) ) ;
#20547=CARTESIAN_POINT ( 'NONE',  ( 52.53356816583844591, 11.72490539043803004, 18.97181229448534268 ) ) ;
#20555=CARTESIAN_POINT ( 'NONE',  ( 59.53125000000000000, 11.65685424949239923, 18.99999999999998934 ) ) ;
#20558=AXIS2_PLACEMENT_3D ( 'NONE', #13369, #15288, #22560 ) ;
#20600=CARTESIAN_POINT ( 'NONE',  ( 56.06250000000000000, 5.999999999999996447, 15.00000000000001599 ) ) ;
#20609=CARTESIAN_POINT ( 'NONE',  ( 53.81250000000000711, 13.00000000000000000, 14.99999999999998757 ) ) ;
#20619=CARTESIAN_POINT ( 'NONE',  ( 57.43518183416157541, 9.931948859054372747, 17.99999999999999645 ) ) ;
#20629=CARTESIAN_POINT ( 'NONE',  ( 57.34143183416159673, 8.689308171935088865, 17.97181229448535689 ) ) ;
#20653=CARTESIAN_POINT ( 'NONE',  ( 57.97106816583845301, 6.971812294485350670, 13.82541045382635403 ) ) ;
#20678=CARTESIAN_POINT ( 'NONE',  ( 54.09375000000000711, 11.65685424949236193, 10.99999999999998401 ) ) ;
#20680=PLANE ( 'NONE',  #17397 ) ;
#20719=CARTESIAN_POINT ( 'NONE',  ( 55.59375000000000711, 11.65685424949236193, 10.99999999999998401 ) ) ;
#20727=CARTESIAN_POINT ( 'NONE',  ( 57.00000000000000000, 12.12132034355963484, 12.87867965644034740 ) ) ;
#20732=CARTESIAN_POINT ( 'NONE',  ( 53.87268183416157541, 7.926799079670491466, 12.83056023321021755 ) ) ;
#20743=CARTESIAN_POINT ( 'NONE',  ( 56.87268183416158962, 7.926799079670491466, 12.83056023321021755 ) ) ;
#20763=CARTESIAN_POINT ( 'NONE',  ( 53.56481816583844591, 6.999999999999998224, 15.06805114094563436 ) ) ;
#20790=CARTESIAN_POINT ( 'NONE',  ( 58.96875000000000711, 5.999999999999987566, 13.34314575050763452 ) ) ;
#20848=CARTESIAN_POINT ( 'NONE',  ( 58.18518183416157541, 10.06805114094562548, 11.99999999999999645 ) ) ;
#20857=CARTESIAN_POINT ( 'NONE',  ( 60.81018183416157541, 12.99999999999999822, 15.06805114094562192 ) ) ;
#20875=CARTESIAN_POINT ( 'NONE',  ( 53.75231816583844591, 7.926799079670502124, 17.16943976678978245 ) ) ;
#20901=CARTESIAN_POINT ( 'NONE',  ( 56.62500000000000000, 12.82842712474620228, 17.82842712474617386 ) ) ;
#20961=CARTESIAN_POINT ( 'NONE',  ( 59.21643183416158962, 12.97181229448535689, 16.31069182806490758 ) ) ;
#20971=CARTESIAN_POINT ( 'NONE',  ( 53.12268183416157541, 12.07320092032950676, 17.16943976678977180 ) ) ;
#20983=CARTESIAN_POINT ( 'NONE',  ( 50.00231816583843170, 12.78030770151603868, 12.12345345202365188 ) ) ;
#20995=CARTESIAN_POINT ( 'NONE',  ( 52.53356816583844591, 11.31069182806492712, 17.97181229448534623 ) ) ;
#21005=SURFACE_STYLE_USAGE ( .BOTH. , #3163 ) ;
#21011=CARTESIAN_POINT ( 'NONE',  ( 52.40625000000000000, 13.99999999999999289, 13.34314575050759544 ) ) ;
#21022=CARTESIAN_POINT ( 'NONE',  ( 58.40625000000000711, 13.99999999999999289, 13.34314575050759544 ) ) ;
#21037=PRODUCT_DEFINITION_CONTEXT ( 'detailed design', #3804, 'design' ) ;
#21063=( BOUNDED_SURFACE ( )  B_SPLINE_SURFACE ( 3, 2, ( 
 ( #17551, #12406, #4836, #12295, #8812, #21107, #23394, #1229, #10384, #1348, #8567, #16110, #6533, #14201, #8460, #4722, #15875, #12531, #6999, #6761, #15767, #3152, #12055, #19321, #8684, #19558, #13962, #23038, #21221, #10496, #15986, #5190, #23273, #21461, #1469, #6881, #12167, #17891, #10619, #2910, #5074, #19671, #10739, #3276, #14318, #3393, #2053, #20018, #3515, #7367, #14562, #16457, #1820, #16222, #3865, #21826, #18124, #1590, #19913, #3981, #23508, #1943, #22173, #11319, #13116, #10848, #7479, #1703, #5787, #5312, #9170, #18237, #21935, #3620, #7122, #14675, #36, #8928, #9047, #148, #18474, #14435, #7246, #11076, #10960, #21701, #5543, #20375, #12875, #22043, #20130, #14795, #5430, #23633, #3736, #11200, #12996 ),
 ( #18362, #9395, #12652, #9282, #14915, #16337, #12766, #16568, #5661, #20260, #16688, #259, #7593, #2418, #4338, #11677, #18594, #13231, #6261, #20961, #9870, #2176, #18946, #13698, #9640, #22654, #2531, #2304, #17165, #19065, #20848, #17289, #7722, #2657, #15035, #16931, #745, #4455, #20619, #15269, #5906, #8080, #13581, #4581, #6149, #11441, #15391, #9513, #18716, #15151, #508, #11794, #18832, #16811, #9999, #7830, #22412, #391, #20497, #22292, #4101, #855, #15501, #6022, #6381, #13350, #8188, #4226, #22771, #11562, #9749, #17047, #22540, #622, #7949, #13472, #20732, #19185, #21082, #10796, #5373, #17403, #17519, #21642, #6618, #2770, #1531, #7312, #23453, #8994, #5131, #1650, #15744, #10228, #14261, #14500, #23577 ),
 ( #12715, #10111, #18070, #12028, #969, #19731, #16397, #10905, #3332, #4694, #7061, #15622, #8301, #16284, #23694, #19292, #14618, #3569, #19967, #21879, #21521, #7185, #12469, #5248, #22891, #11917, #18185, #1086, #2881, #16167, #12595, #6506, #13826, #19853, #1766, #8431, #23013, #10675, #17951, #8873, #14381, #3458, #21764, #9107, #20314, #3915, #20197, #12933, #204, #20079, #9228, #11017, #4161, #13059, #11254, #7885, #21992, #7535, #11507, #16988, #2360, #1884, #18779, #18527, #2114, #14852, #5964, #22107, #5606, #16873, #9449, #5486, #11142, #7657, #16626, #14980, #16745, #16514, #18303, #22348, #9691, #560, #12821, #326, #5727, #22233, #5841, #13168, #13288, #20434, #4043, #11373, #3679, #89, #450, #15204, #18651 ),
 ( #3806, #9580, #2240, #18416, #7775, #20555, #15093, #7423, #14733, #1995, #9336, #20790, #4637, #1028, #802, #19127, #9807, #21022, #17465, #8489, #10054, #15330, #22827, #6079, #22600, #18998, #4396, #15565, #6442, #17229, #11735, #674, #6204, #11851, #13762, #19351, #20901, #11971, #15682, #17344, #2587, #8364, #22955, #4282, #9932, #17098, #1148, #8009, #15445, #10174, #6563, #8134, #13522, #4514, #22712, #13638, #6323, #13411, #13879, #2713, #911, #22468, #8247, #20678, #11616, #19237, #2940, #18886, #10291, #2827, #21137, #4750, #17582, #2472, #12086, #8713, #12436, #17807, #6676, #21491, #16019, #23065, #1257, #14350, #8963, #21251, #21374, #1507, #10529, #13989, #5104, #10877, #3304, #12563, #23308, #5218, #19587 ),
 ( #3429, #10647, #19701, #4995, #17922, #16253, #4868, #8846, #7152, #16141, #5344, #21611, #12203, #23426, #7033, #8596, #19823, #12324, #10770, #23544, #19474, #14466, #1375, #3183, #18044, #6917, #21732, #3072, #1621, #15902, #10416, #14234, #19942, #12688, #3542, #23179, #18153, #17696, #6790, #1737, #15793, #14111, #4132, #421, #9547, #11474, #18388, #5813, #11110, #18499, #16367, #20524, #16843, #21962, #16486, #13028, #2084, #9076, #14593, #9425, #2208, #18750, #7280, #7394, #12795, #21853, #23663, #16714, #10987, #5693, #177, #7509, #62, #14706, #3770, #5459, #20047, #3651, #7748, #16598, #14822, #18266, #1851, #1968, #15063, #9200, #5934, #5575, #22319, #22074, #20288, #9308, #13261, #3889, #12902, #20404, #11225 ),
 ( #292, #20163, #7627, #14950, #22202, #13140, #4011, #11349, #18621, #18859, #2333, #20653, #4726, #16957, #2691, #22926, #12059, #13855, #4257, #8219, #2445, #6538, #6052, #2557, #18974, #22682, #4368, #534, #8111, #9905, #9667, #11591, #885, #19214, #7856, #15180, #7982, #4484, #13500, #11823, #15420, #13384, #22439, #2803, #9779, #6295, #10145, #17437, #13731, #1003, #21110, #17075, #778, #17200, #649, #13612, #20875, #19099, #20763, #15302, #15536, #22576, #6180, #11706, #10031, #17319, #22802, #6416, #8336, #20995, #4615, #11949, #15654, #23041, #10744, #21463, #8931, #17895, #2913, #5076, #1351, #4839, #23396, #15877, #8686, #19797, #1120, #18017, #4966, #6764, #12408, #14080, #3395, #17554, #1472, #19442, #8465 ),
 ( #3154, #12172, #14205, #6652, #15769, #16113, #23510, #3040, #14437, #1592, #16224, #21705, #12298, #7001, #21342, #19673, #10263, #7125, #5314, #8570, #10389, #23275, #3278, #19325, #13965, #10621, #12533, #21226, #17670, #1231, #23152, #19560, #10499, #8815, #17779, #15991, #6884, #14320, #21579, #5192, #7370, #3517, #16339, #18127, #11323, #20132, #11079, #15037, #5433, #14679, #18596, #393, #9518, #9049, #2179, #18365, #1946, #21937, #13118, #5545, #12768, #262, #9284, #20377, #12878, #14566, #16572, #1824, #3740, #151, #10850, #14919, #9173, #20020, #12656, #7248, #22294, #1705, #12997, #16814, #19917, #7724, #21830, #18476, #3623, #23637, #10962, #7481, #14797, #22046, #5665, #18239, #20263, #3868, #16460, #39, #11202 ) ),
 .UNSPECIFIED., .T., .F., .F. ) 
 B_SPLINE_SURFACE_WITH_KNOTS ( ( 4, 3, 4 ),
 ( 3, 2, 2, 2, 2, 2, 2, 2, 2, 2, 2, 2, 2, 2, 2, 2, 2, 2, 2, 2, 2, 2, 2, 2, 2, 2, 2, 2, 2, 2, 2, 2, 2, 2, 2, 2, 2, 2, 2, 2, 2, 2, 2, 2, 2, 2, 2, 2, 3 ),
 ( 0.000000000000000000, 0.5000000000000000000, 1.000000000000000000 ),
 ( 0.000000000000000000, 0.02083333333333333218, 0.04166666666666666435, 0.06250000000000000000, 0.08333333333333332871, 0.1041666666666666713, 0.1250000000000000000, 0.1458333333333333426, 0.1666666666666666574, 0.1875000000000000000, 0.2083333333333333426, 0.2291666666666666574, 0.2500000000000000000, 0.2708333333333333148, 0.2916666666666666852, 0.3125000000000000000, 0.3333333333333333148, 0.3541666666666666852, 0.3750000000000000000, 0.3958333333333333148, 0.4166666666666666852, 0.4375000000000000000, 0.4583333333333333148, 0.4791666666666666852, 0.5000000000000000000, 0.5208333333333333703, 0.5416666666666666297, 0.5625000000000000000, 0.5833333333333333703, 0.6041666666666666297, 0.6250000000000000000, 0.6458333333333333703, 0.6666666666666666297, 0.6875000000000000000, 0.7083333333333333703, 0.7291666666666666297, 0.7500000000000000000, 0.7708333333333333703, 0.7916666666666666297, 0.8125000000000000000, 0.8333333333333333703, 0.8541666666666666297, 0.8750000000000000000, 0.8958333333333333703, 0.9166666666666666297, 0.9375000000000000000, 0.9583333333333333703, 0.9791666666666666297, 1.000000000000000000 ),
 .UNSPECIFIED. ) 
 GEOMETRIC_REPRESENTATION_ITEM ( )  RATIONAL_B_SPLINE_SURFACE ( (
 ( 1.000000000000000000, 0.9238795325112867385, 1.000000000000000000, 0.9238795325112867385, 1.000000000000000000, 0.9238795325112867385, 1.000000000000000000, 0.9238795325112867385, 1.000000000000000000, 0.9238795325112867385, 1.000000000000000000, 0.9238795325112867385, 1.000000000000000000, 0.9238795325112867385, 1.000000000000000000, 0.9238795325112867385, 1.000000000000000000, 0.9238795325112867385, 1.000000000000000000, 0.9238795325112867385, 1.000000000000000000, 0.9238795325112867385, 1.000000000000000000, 0.9238795325112867385, 1.000000000000000000, 0.9238795325112867385, 1.000000000000000000, 0.9238795325112867385, 1.000000000000000000, 0.9238795325112867385, 1.000000000000000000, 0.9238795325112867385, 1.000000000000000000, 0.9238795325112867385, 1.000000000000000000, 0.9238795325112867385, 1.000000000000000000, 0.9238795325112867385, 1.000000000000000000, 0.9238795325112867385, 1.000000000000000000, 0.9238795325112867385, 1.000000000000000000, 0.9238795325112867385, 1.000000000000000000, 0.9238795325112867385, 1.000000000000000000, 0.9238795325112867385, 1.000000000000000000, 0.9238795325112867385, 1.000000000000000000, 0.9238795325112867385, 1.000000000000000000, 0.9238795325112867385, 1.000000000000000000, 0.9238795325112867385, 1.000000000000000000, 0.9238795325112867385, 1.000000000000000000, 0.9238795325112867385, 1.000000000000000000, 0.9238795325112867385, 1.000000000000000000, 0.9238795325112867385, 1.000000000000000000, 0.9238795325112867385, 1.000000000000000000, 0.9238795325112867385, 1.000000000000000000, 0.9238795325112867385, 1.000000000000000000, 0.9238795325112867385, 1.000000000000000000, 0.9238795325112867385, 1.000000000000000000, 0.9238795325112867385, 1.000000000000000000, 0.9238795325112867385, 1.000000000000000000, 0.9238795325112867385, 1.000000000000000000, 0.9238795325112867385, 1.000000000000000000, 0.9238795325112867385, 1.000000000000000000, 0.9238795325112867385, 1.000000000000000000, 0.9238795325112867385, 1.000000000000000000, 0.9238795325112867385, 1.000000000000000000, 0.9238795325112867385, 1.000000000000000000, 0.9238795325112867385, 1.000000000000000000, 0.9238795325112867385, 1.000000000000000000),
 ( 0.3333333333333333703, 0.3079598441704289313, 0.3333333333333333703, 0.3079598441704289313, 0.3333333333333333703, 0.3079598441704289313, 0.3333333333333333703, 0.3079598441704289313, 0.3333333333333333703, 0.3079598441704289313, 0.3333333333333333703, 0.3079598441704289313, 0.3333333333333333703, 0.3079598441704289313, 0.3333333333333333703, 0.3079598441704289313, 0.3333333333333333703, 0.3079598441704289313, 0.3333333333333333703, 0.3079598441704289313, 0.3333333333333333703, 0.3079598441704289313, 0.3333333333333333703, 0.3079598441704289313, 0.3333333333333333703, 0.3079598441704289313, 0.3333333333333333703, 0.3079598441704289313, 0.3333333333333333703, 0.3079598441704289313, 0.3333333333333333703, 0.3079598441704289313, 0.3333333333333333703, 0.3079598441704289313, 0.3333333333333333703, 0.3079598441704289313, 0.3333333333333333703, 0.3079598441704289313, 0.3333333333333333703, 0.3079598441704289313, 0.3333333333333333703, 0.3079598441704289313, 0.3333333333333333703, 0.3079598441704289313, 0.3333333333333333703, 0.3079598441704289313, 0.3333333333333333703, 0.3079598441704289313, 0.3333333333333333703, 0.3079598441704289313, 0.3333333333333333703, 0.3079598441704289313, 0.3333333333333333703, 0.3079598441704289313, 0.3333333333333333703, 0.3079598441704289313, 0.3333333333333333703, 0.3079598441704289313, 0.3333333333333333703, 0.3079598441704289313, 0.3333333333333333703, 0.3079598441704289313, 0.3333333333333333703, 0.3079598441704289313, 0.3333333333333333703, 0.3079598441704289313, 0.3333333333333333703, 0.3079598441704289313, 0.3333333333333333703, 0.3079598441704289313, 0.3333333333333333703, 0.3079598441704289313, 0.3333333333333333703, 0.3079598441704289313, 0.3333333333333333703, 0.3079598441704289313, 0.3333333333333333703, 0.3079598441704289313, 0.3333333333333333703, 0.3079598441704289313, 0.3333333333333333703, 0.3079598441704289313, 0.3333333333333333703, 0.3079598441704289313, 0.3333333333333333703, 0.3079598441704289313, 0.3333333333333333703, 0.3079598441704289313, 0.3333333333333333703, 0.3079598441704289313, 0.3333333333333333703, 0.3079598441704289313, 0.3333333333333333703, 0.3079598441704289313, 0.3333333333333333703, 0.3079598441704289313, 0.3333333333333333703),
 ( 0.3333333333333333703, 0.3079598441704289313, 0.3333333333333333703, 0.3079598441704289313, 0.3333333333333333703, 0.3079598441704289313, 0.3333333333333333703, 0.3079598441704289313, 0.3333333333333333703, 0.3079598441704289313, 0.3333333333333333703, 0.3079598441704289313, 0.3333333333333333703, 0.3079598441704289313, 0.3333333333333333703, 0.3079598441704289313, 0.3333333333333333703, 0.3079598441704289313, 0.3333333333333333703, 0.3079598441704289313, 0.3333333333333333703, 0.3079598441704289313, 0.3333333333333333703, 0.3079598441704289313, 0.3333333333333333703, 0.3079598441704289313, 0.3333333333333333703, 0.3079598441704289313, 0.3333333333333333703, 0.3079598441704289313, 0.3333333333333333703, 0.3079598441704289313, 0.3333333333333333703, 0.3079598441704289313, 0.3333333333333333703, 0.3079598441704289313, 0.3333333333333333703, 0.3079598441704289313, 0.3333333333333333703, 0.3079598441704289313, 0.3333333333333333703, 0.3079598441704289313, 0.3333333333333333703, 0.3079598441704289313, 0.3333333333333333703, 0.3079598441704289313, 0.3333333333333333703, 0.3079598441704289313, 0.3333333333333333703, 0.3079598441704289313, 0.3333333333333333703, 0.3079598441704289313, 0.3333333333333333703, 0.3079598441704289313, 0.3333333333333333703, 0.3079598441704289313, 0.3333333333333333703, 0.3079598441704289313, 0.3333333333333333703, 0.3079598441704289313, 0.3333333333333333703, 0.3079598441704289313, 0.3333333333333333703, 0.3079598441704289313, 0.3333333333333333703, 0.3079598441704289313, 0.3333333333333333703, 0.3079598441704289313, 0.3333333333333333703, 0.3079598441704289313, 0.3333333333333333703, 0.3079598441704289313, 0.3333333333333333703, 0.3079598441704289313, 0.3333333333333333703, 0.3079598441704289313, 0.3333333333333333703, 0.3079598441704289313, 0.3333333333333333703, 0.3079598441704289313, 0.3333333333333333703, 0.3079598441704289313, 0.3333333333333333703, 0.3079598441704289313, 0.3333333333333333703, 0.3079598441704289313, 0.3333333333333333703, 0.3079598441704289313, 0.3333333333333333703, 0.3079598441704289313, 0.3333333333333333703, 0.3079598441704289313, 0.3333333333333333703, 0.3079598441704289313, 0.3333333333333333703, 0.3079598441704289313, 0.3333333333333333703),
 ( 1.000000000000000000, 0.9238795325112867385, 1.000000000000000000, 0.9238795325112867385, 1.000000000000000000, 0.9238795325112867385, 1.000000000000000000, 0.9238795325112867385, 1.000000000000000000, 0.9238795325112867385, 1.000000000000000000, 0.9238795325112867385, 1.000000000000000000, 0.9238795325112867385, 1.000000000000000000, 0.9238795325112867385, 1.000000000000000000, 0.9238795325112867385, 1.000000000000000000, 0.9238795325112867385, 1.000000000000000000, 0.9238795325112867385, 1.000000000000000000, 0.9238795325112867385, 1.000000000000000000, 0.9238795325112867385, 1.000000000000000000, 0.9238795325112867385, 1.000000000000000000, 0.9238795325112867385, 1.000000000000000000, 0.9238795325112867385, 1.000000000000000000, 0.9238795325112867385, 1.000000000000000000, 0.9238795325112867385, 1.000000000000000000, 0.9238795325112867385, 1.000000000000000000, 0.9238795325112867385, 1.000000000000000000, 0.9238795325112867385, 1.000000000000000000, 0.9238795325112867385, 1.000000000000000000, 0.9238795325112867385, 1.000000000000000000, 0.9238795325112867385, 1.000000000000000000, 0.9238795325112867385, 1.000000000000000000, 0.9238795325112867385, 1.000000000000000000, 0.9238795325112867385, 1.000000000000000000, 0.9238795325112867385, 1.000000000000000000, 0.9238795325112867385, 1.000000000000000000, 0.9238795325112867385, 1.000000000000000000, 0.9238795325112867385, 1.000000000000000000, 0.9238795325112867385, 1.000000000000000000, 0.9238795325112867385, 1.000000000000000000, 0.9238795325112867385, 1.000000000000000000, 0.9238795325112867385, 1.000000000000000000, 0.9238795325112867385, 1.000000000000000000, 0.9238795325112867385, 1.000000000000000000, 0.9238795325112867385, 1.000000000000000000, 0.9238795325112867385, 1.000000000000000000, 0.9238795325112867385, 1.000000000000000000, 0.9238795325112867385, 1.000000000000000000, 0.9238795325112867385, 1.000000000000000000, 0.9238795325112867385, 1.000000000000000000, 0.9238795325112867385, 1.000000000000000000, 0.9238795325112867385, 1.000000000000000000, 0.9238795325112867385, 1.000000000000000000, 0.9238795325112867385, 1.000000000000000000, 0.9238795325112867385, 1.000000000000000000),
 ( 0.3333333333333333703, 0.3079598441704289313, 0.3333333333333333703, 0.3079598441704289313, 0.3333333333333333703, 0.3079598441704289313, 0.3333333333333333703, 0.3079598441704289313, 0.3333333333333333703, 0.3079598441704289313, 0.3333333333333333703, 0.3079598441704289313, 0.3333333333333333703, 0.3079598441704289313, 0.3333333333333333703, 0.3079598441704289313, 0.3333333333333333703, 0.3079598441704289313, 0.3333333333333333703, 0.3079598441704289313, 0.3333333333333333703, 0.3079598441704289313, 0.3333333333333333703, 0.3079598441704289313, 0.3333333333333333703, 0.3079598441704289313, 0.3333333333333333703, 0.3079598441704289313, 0.3333333333333333703, 0.3079598441704289313, 0.3333333333333333703, 0.3079598441704289313, 0.3333333333333333703, 0.3079598441704289313, 0.3333333333333333703, 0.3079598441704289313, 0.3333333333333333703, 0.3079598441704289313, 0.3333333333333333703, 0.3079598441704289313, 0.3333333333333333703, 0.3079598441704289313, 0.3333333333333333703, 0.3079598441704289313, 0.3333333333333333703, 0.3079598441704289313, 0.3333333333333333703, 0.3079598441704289313, 0.3333333333333333703, 0.3079598441704289313, 0.3333333333333333703, 0.3079598441704289313, 0.3333333333333333703, 0.3079598441704289313, 0.3333333333333333703, 0.3079598441704289313, 0.3333333333333333703, 0.3079598441704289313, 0.3333333333333333703, 0.3079598441704289313, 0.3333333333333333703, 0.3079598441704289313, 0.3333333333333333703, 0.3079598441704289313, 0.3333333333333333703, 0.3079598441704289313, 0.3333333333333333703, 0.3079598441704289313, 0.3333333333333333703, 0.3079598441704289313, 0.3333333333333333703, 0.3079598441704289313, 0.3333333333333333703, 0.3079598441704289313, 0.3333333333333333703, 0.3079598441704289313, 0.3333333333333333703, 0.3079598441704289313, 0.3333333333333333703, 0.3079598441704289313, 0.3333333333333333703, 0.3079598441704289313, 0.3333333333333333703, 0.3079598441704289313, 0.3333333333333333703, 0.3079598441704289313, 0.3333333333333333703, 0.3079598441704289313, 0.3333333333333333703, 0.3079598441704289313, 0.3333333333333333703, 0.3079598441704289313, 0.3333333333333333703, 0.3079598441704289313, 0.3333333333333333703, 0.3079598441704289313, 0.3333333333333333703),
 ( 0.3333333333333333703, 0.3079598441704289313, 0.3333333333333333703, 0.3079598441704289313, 0.3333333333333333703, 0.3079598441704289313, 0.3333333333333333703, 0.3079598441704289313, 0.3333333333333333703, 0.3079598441704289313, 0.3333333333333333703, 0.3079598441704289313, 0.3333333333333333703, 0.3079598441704289313, 0.3333333333333333703, 0.3079598441704289313, 0.3333333333333333703, 0.3079598441704289313, 0.3333333333333333703, 0.3079598441704289313, 0.3333333333333333703, 0.3079598441704289313, 0.3333333333333333703, 0.3079598441704289313, 0.3333333333333333703, 0.3079598441704289313, 0.3333333333333333703, 0.3079598441704289313, 0.3333333333333333703, 0.3079598441704289313, 0.3333333333333333703, 0.3079598441704289313, 0.3333333333333333703, 0.3079598441704289313, 0.3333333333333333703, 0.3079598441704289313, 0.3333333333333333703, 0.3079598441704289313, 0.3333333333333333703, 0.3079598441704289313, 0.3333333333333333703, 0.3079598441704289313, 0.3333333333333333703, 0.3079598441704289313, 0.3333333333333333703, 0.3079598441704289313, 0.3333333333333333703, 0.3079598441704289313, 0.3333333333333333703, 0.3079598441704289313, 0.3333333333333333703, 0.3079598441704289313, 0.3333333333333333703, 0.3079598441704289313, 0.3333333333333333703, 0.3079598441704289313, 0.3333333333333333703, 0.3079598441704289313, 0.3333333333333333703, 0.3079598441704289313, 0.3333333333333333703, 0.3079598441704289313, 0.3333333333333333703, 0.3079598441704289313, 0.3333333333333333703, 0.3079598441704289313, 0.3333333333333333703, 0.3079598441704289313, 0.3333333333333333703, 0.3079598441704289313, 0.3333333333333333703, 0.3079598441704289313, 0.3333333333333333703, 0.3079598441704289313, 0.3333333333333333703, 0.3079598441704289313, 0.3333333333333333703, 0.3079598441704289313, 0.3333333333333333703, 0.3079598441704289313, 0.3333333333333333703, 0.3079598441704289313, 0.3333333333333333703, 0.3079598441704289313, 0.3333333333333333703, 0.3079598441704289313, 0.3333333333333333703, 0.3079598441704289313, 0.3333333333333333703, 0.3079598441704289313, 0.3333333333333333703, 0.3079598441704289313, 0.3333333333333333703, 0.3079598441704289313, 0.3333333333333333703, 0.3079598441704289313, 0.3333333333333333703),
 ( 1.000000000000000000, 0.9238795325112867385, 1.000000000000000000, 0.9238795325112867385, 1.000000000000000000, 0.9238795325112867385, 1.000000000000000000, 0.9238795325112867385, 1.000000000000000000, 0.9238795325112867385, 1.000000000000000000, 0.9238795325112867385, 1.000000000000000000, 0.9238795325112867385, 1.000000000000000000, 0.9238795325112867385, 1.000000000000000000, 0.9238795325112867385, 1.000000000000000000, 0.9238795325112867385, 1.000000000000000000, 0.9238795325112867385, 1.000000000000000000, 0.9238795325112867385, 1.000000000000000000, 0.9238795325112867385, 1.000000000000000000, 0.9238795325112867385, 1.000000000000000000, 0.9238795325112867385, 1.000000000000000000, 0.9238795325112867385, 1.000000000000000000, 0.9238795325112867385, 1.000000000000000000, 0.9238795325112867385, 1.000000000000000000, 0.9238795325112867385, 1.000000000000000000, 0.9238795325112867385, 1.000000000000000000, 0.9238795325112867385, 1.000000000000000000, 0.9238795325112867385, 1.000000000000000000, 0.9238795325112867385, 1.000000000000000000, 0.9238795325112867385, 1.000000000000000000, 0.9238795325112867385, 1.000000000000000000, 0.9238795325112867385, 1.000000000000000000, 0.9238795325112867385, 1.000000000000000000, 0.9238795325112867385, 1.000000000000000000, 0.9238795325112867385, 1.000000000000000000, 0.9238795325112867385, 1.000000000000000000, 0.9238795325112867385, 1.000000000000000000, 0.9238795325112867385, 1.000000000000000000, 0.9238795325112867385, 1.000000000000000000, 0.9238795325112867385, 1.000000000000000000, 0.9238795325112867385, 1.000000000000000000, 0.9238795325112867385, 1.000000000000000000, 0.9238795325112867385, 1.000000000000000000, 0.9238795325112867385, 1.000000000000000000, 0.9238795325112867385, 1.000000000000000000, 0.9238795325112867385, 1.000000000000000000, 0.9238795325112867385, 1.000000000000000000, 0.9238795325112867385, 1.000000000000000000, 0.9238795325112867385, 1.000000000000000000, 0.9238795325112867385, 1.000000000000000000, 0.9238795325112867385, 1.000000000000000000, 0.9238795325112867385, 1.000000000000000000, 0.9238795325112867385, 1.000000000000000000, 0.9238795325112867385, 1.000000000000000000) ) ) 
 REPRESENTATION_ITEM ( '' )  SURFACE ( )  );
#21082=CARTESIAN_POINT ( 'NONE',  ( 53.68518183416157541, 10.06805114094562548, 11.99999999999999645 ) ) ;
#21092=CARTESIAN_POINT ( 'NONE',  ( 58.56018183416157541, 5.999999999999996447, 14.93194885905437808 ) ) ;
#21101=CARTESIAN_POINT ( 'NONE',  ( 55.34606816583843880, 8.825410453826357582, 18.02818770551464667 ) ) ;
#21107=CARTESIAN_POINT ( 'NONE',  ( 59.53125000000000000, 11.24264068711929276, 18.00000000000000355 ) ) ;
#21110=CARTESIAN_POINT ( 'NONE',  ( 54.31481816583844591, 12.99999999999999822, 14.93194885905435676 ) ) ;
#21120=FACE_OUTER_BOUND ( 'NONE', #13773, .T. ) ;
#21128=DIRECTION ( 'NONE',  ( 1.000000000000000000, 0.000000000000000000, -0.000000000000000000 ) ) ;
#21137=CARTESIAN_POINT ( 'NONE',  ( 53.43750000000000711, 10.00000000000001776, 18.99999999999999645 ) ) ;
#21193=CARTESIAN_POINT ( 'NONE',  ( 60.00000000000005684, 13.04144815258546330, 15.11939319870875309 ) ) ;
#21204=CARTESIAN_POINT ( 'NONE',  ( 54.34143183416158251, 8.689308171935088865, 17.97181229448535689 ) ) ;
#21214=CARTESIAN_POINT ( 'NONE',  ( 51.03356816583844591, 11.72490539043803004, 18.97181229448534268 ) ) ;
#21221=CARTESIAN_POINT ( 'NONE',  ( 57.37500000000000000, 7.878679656440349177, 12.87867965644035984 ) ) ;
#21225=CARTESIAN_POINT ( 'NONE',  ( 60.00000000000000711, 12.12132034355963484, 12.87867965644034740 ) ) ;
#21226=CARTESIAN_POINT ( 'NONE',  ( 57.46875000000000711, 6.999999999999992895, 13.75735931288071967 ) ) ;
#21251=CARTESIAN_POINT ( 'NONE',  ( 52.03124999999999289, 11.65685424949239923, 18.99999999999998934 ) ) ;
#21267=CARTESIAN_POINT ( 'NONE',  ( 52.59375000000000711, 11.65685424949236193, 10.99999999999998401 ) ) ;
#21299=CARTESIAN_POINT ( 'NONE',  ( 52.12500000000000711, 12.12132034355964727, 17.12132034355963484 ) ) ;
#21307=CARTESIAN_POINT ( 'NONE',  ( 60.00000000000003553, 13.00089921235714741, 17.44255260030195842 ) ) ;
#21320=CARTESIAN_POINT ( 'NONE',  ( 54.43518183416157541, 9.931948859054372747, 17.99999999999999645 ) ) ;
#21332=CARTESIAN_POINT ( 'NONE',  ( 50.09606816583843880, 11.58880310854672935, 10.97181229448534445 ) ) ;
#21342=CARTESIAN_POINT ( 'NONE',  ( 58.68750000000000000, 9.999999999999989342, 11.99999999999999467 ) ) ;
#21353=CARTESIAN_POINT ( 'NONE',  ( 59.62500000000000711, 12.12132034355964727, 17.12132034355963484 ) ) ;
#21374=CARTESIAN_POINT ( 'NONE',  ( 51.93750000000000711, 10.00000000000001776, 18.99999999999999645 ) ) ;
#21396=CARTESIAN_POINT ( 'NONE',  ( 51.00000000000000711, 12.82842712474617741, 12.17157287525379239 ) ) ;
#21413=CARTESIAN_POINT ( 'NONE',  ( 58.21875000000000711, 13.00000000000000533, 16.24264068711927322 ) ) ;
#21433=CARTESIAN_POINT ( 'NONE',  ( 60.00000000000002132, 11.14543721897689110, 18.43906226982675634 ) ) ;
#21443=CARTESIAN_POINT ( 'NONE',  ( 60.34143183416158962, 8.275094609562001935, 18.97181229448536044 ) ) ;
#21453=CARTESIAN_POINT ( 'NONE',  ( 58.34606816583844591, 8.825410453826357582, 18.02818770551464667 ) ) ;
#21461=CARTESIAN_POINT ( 'NONE',  ( 56.90625000000000711, 12.99999999999999645, 13.75735931288070191 ) ) ;
#21463=CARTESIAN_POINT ( 'NONE',  ( 51.97106816583844591, 6.971812294485350670, 13.82541045382635403 ) ) ;
#21491=CARTESIAN_POINT ( 'NONE',  ( 52.59375000000000711, 11.65685424949236193, 10.99999999999998401 ) ) ;
#21498=EDGE_CURVE ( 'NONE', #1478, #8676, #4160, .T. ) ;
#21511=CARTESIAN_POINT ( 'NONE',  ( 52.31250000000000711, 14.00000000000000000, 14.99999999999997691 ) ) ;
#21521=CARTESIAN_POINT ( 'NONE',  ( 59.12268183416157541, 12.78030770151606177, 17.87654654797631792 ) ) ;
#21531=CARTESIAN_POINT ( 'NONE',  ( 55.12500000000000711, 12.12132034355964727, 17.12132034355963484 ) ) ;
#21551=CARTESIAN_POINT ( 'NONE',  ( 60.00000000000000711, 11.02697561308437812, 18.23285838809245618 ) ) ;
#21560=CARTESIAN_POINT ( 'NONE',  ( 57.99768183416157541, 12.87654654797631792, 12.21969229848393113 ) ) ;
#21569=CARTESIAN_POINT ( 'NONE',  ( 51.68981816583844591, 9.931948859054354983, 11.99999999999999645 ) ) ;
#21579=CARTESIAN_POINT ( 'NONE',  ( 56.43750000000000000, 10.00000000000000711, 17.99999999999999645 ) ) ;
#21588=CARTESIAN_POINT ( 'NONE',  ( 57.75000000000000000, 7.878679656440361612, 17.12132034355964549 ) ) ;
#21611=CARTESIAN_POINT ( 'NONE',  ( 57.97106816583845301, 5.971812294485345340, 13.41119689145326710 ) ) ;
#21613=FILL_AREA_STYLE_COLOUR ( '', #9552 ) ;
#21633=CARTESIAN_POINT ( 'NONE',  ( 55.31250000000000711, 14.00000000000000000, 14.99999999999997691 ) ) ;
#21642=CARTESIAN_POINT ( 'NONE',  ( 53.21643183416158251, 12.97181229448535689, 16.31069182806490758 ) ) ;
#21649=CARTESIAN_POINT ( 'NONE',  ( 55.87500000000000711, 7.878679656440349177, 12.87867965644035984 ) ) ;
#21672=CARTESIAN_POINT ( 'NONE',  ( 60.00000000000000000, 13.97680642442999854, 14.92529509588244352 ) ) ;
#21684=CARTESIAN_POINT ( 'NONE',  ( 53.40393183416157541, 14.02818770551463956, 13.41119689145323335 ) ) ;
#21695=CARTESIAN_POINT ( 'NONE',  ( 59.06250000000000711, 6.999999999999997335, 15.00000000000000533 ) ) ;
#21701=CARTESIAN_POINT ( 'NONE',  ( 52.03124999999999289, 11.24264068711929276, 18.00000000000000355 ) ) ;
#21705=CARTESIAN_POINT ( 'NONE',  ( 58.96875000000000711, 6.999999999999992895, 13.75735931288071967 ) ) ;
#21712=CARTESIAN_POINT ( 'NONE',  ( 52.78125000000000711, 8.757359312880703683, 11.99999999999999822 ) ) ;
#21732=CARTESIAN_POINT ( 'NONE',  ( 56.56481816583843170, 5.999999999999996447, 15.06805114094564502 ) ) ;
#21747=CARTESIAN_POINT ( 'NONE',  ( 56.81250000000000000, 14.00000000000000000, 14.99999999999997691 ) ) ;
#21752=CARTESIAN_POINT ( 'NONE',  ( 53.25000000000000711, 7.171572875253819923, 17.82842712474619873 ) ) ;
#21764=CARTESIAN_POINT ( 'NONE',  ( 57.06018183416157541, 5.999999999999996447, 14.93194885905437808 ) ) ;
#21773=CARTESIAN_POINT ( 'NONE',  ( 54.18750000000000711, 9.999999999999989342, 11.99999999999999467 ) ) ;
#21812=CARTESIAN_POINT ( 'NONE',  ( 53.68518183416157541, 10.06805114094561659, 10.99999999999999645 ) ) ;
#21821=CARTESIAN_POINT ( 'NONE',  ( 50.93981816583844591, 10.06805114094563791, 17.99999999999999645 ) ) ;
#21826=CARTESIAN_POINT ( 'NONE',  ( 54.84375000000000000, 8.757359312880723223, 18.00000000000000355 ) ) ;
#21830=CARTESIAN_POINT ( 'NONE',  ( 52.31250000000000711, 13.00000000000000000, 14.99999999999998757 ) ) ;
#21839=CARTESIAN_POINT ( 'NONE',  ( 53.62500000000000711, 12.12132034355964727, 17.12132034355963484 ) ) ;
#21853=CARTESIAN_POINT ( 'NONE',  ( 52.90856816583843880, 13.97181229448534978, 13.27509460956196641 ) ) ;
#21866=CARTESIAN_POINT ( 'NONE',  ( 54.18750000000000711, 9.999999999999978684, 10.99999999999999645 ) ) ;
#21870=CARTESIAN_POINT ( 'NONE',  ( 53.18981816583844591, 9.931948859054346102, 10.99999999999999467 ) ) ;
#21879=CARTESIAN_POINT ( 'NONE',  ( 59.21643183416158962, 13.97181229448536399, 16.72490539043799629 ) ) ;
#21886=CARTESIAN_POINT ( 'NONE',  ( 55.21875000000000711, 13.00000000000000533, 16.24264068711927322 ) ) ;
#21916=CARTESIAN_POINT ( 'NONE',  ( 53.77893183416158251, 8.411196891453236901, 10.97181229448535511 ) ) ;
#21926=CARTESIAN_POINT ( 'NONE',  ( 54.59606816583844591, 11.17458954617364242, 11.97181229448534800 ) ) ;
#21935=CARTESIAN_POINT ( 'NONE',  ( 53.25000000000000711, 7.878679656440361612, 17.12132034355964549 ) ) ;
#21937=CARTESIAN_POINT ( 'NONE',  ( 54.65625000000001421, 7.000000000000003553, 16.24264068711929099 ) ) ;
#21944=CARTESIAN_POINT ( 'NONE',  ( 53.43750000000000711, 10.00000000000000711, 17.99999999999999645 ) ) ;
#21962=CARTESIAN_POINT ( 'NONE',  ( 54.03356816583844591, 11.72490539043803004, 18.97181229448534268 ) ) ;
#21977=CARTESIAN_POINT ( 'NONE',  ( 55.21875000000000711, 14.00000000000001066, 16.65685424949235482 ) ) ;
#21981=CARTESIAN_POINT ( 'NONE',  ( 52.72106816583844591, 14.02818770551465377, 16.58880310854672757 ) ) ;
#21992=CARTESIAN_POINT ( 'NONE',  ( 55.74768183416157541, 7.123453452023678523, 17.78030770151605822 ) ) ;
#22029=CARTESIAN_POINT ( 'NONE',  ( 57.52893183416158962, 11.58880310854676132, 19.02818770551463956 ) ) ;
#22037=CARTESIAN_POINT ( 'NONE',  ( 53.56481816583844591, 6.999999999999998224, 15.06805114094563436 ) ) ;
#22043=CARTESIAN_POINT ( 'NONE',  ( 51.65625000000000711, 7.000000000000003553, 16.24264068711929099 ) ) ;
#22046=CARTESIAN_POINT ( 'NONE',  ( 51.65625000000000711, 7.000000000000003553, 16.24264068711929099 ) ) ;
#22055=CARTESIAN_POINT ( 'NONE',  ( 51.75000000000000711, 7.878679656440361612, 17.12132034355964549 ) ) ;
#22074=CARTESIAN_POINT ( 'NONE',  ( 50.65856816583843880, 6.028187705514649330, 16.72490539043803182 ) ) ;
#22093=CARTESIAN_POINT ( 'NONE',  ( 56.34375000000000711, 8.343145750507636293, 19.00000000000000000 ) ) ;
#22097=CARTESIAN_POINT ( 'NONE',  ( 55.81481816583843170, 14.00000000000000178, 14.93194885905434610 ) ) ;
#22107=CARTESIAN_POINT ( 'NONE',  ( 54.71643183416158251, 13.97181229448536399, 16.72490539043799629 ) ) ;
#22155=CARTESIAN_POINT ( 'NONE',  ( 57.09375000000000711, 11.65685424949236193, 10.99999999999998401 ) ) ;
#22164=CARTESIAN_POINT ( 'NONE',  ( 56.53125000000000711, 11.24264068711929276, 18.00000000000000355 ) ) ;
#22173=CARTESIAN_POINT ( 'NONE',  ( 54.18750000000000711, 9.999999999999989342, 11.99999999999999467 ) ) ;
#22184=CARTESIAN_POINT ( 'NONE',  ( 55.31250000000000711, 13.00000000000000000, 14.99999999999998757 ) ) ;
#22202=CARTESIAN_POINT ( 'NONE',  ( 58.62731816583843170, 12.16943976678978601, 17.07320092032949432 ) ) ;
#22217=CARTESIAN_POINT ( 'NONE',  ( 53.15625000000000711, 6.000000000000004441, 16.65685424949239390 ) ) ;
#22221=CARTESIAN_POINT ( 'NONE',  ( 56.47106816583845301, 5.971812294485345340, 13.41119689145326710 ) ) ;
#22233=CARTESIAN_POINT ( 'NONE',  ( 53.02893183416157541, 11.58880310854676132, 19.02818770551463956 ) ) ;
#22241=CARTESIAN_POINT ( 'NONE',  ( 53.43750000000000711, 10.00000000000000711, 17.99999999999999645 ) ) ;
#22276=CARTESIAN_POINT ( 'NONE',  ( 52.18518183416157541, 10.06805114094561659, 10.99999999999999645 ) ) ;
#22283=CARTESIAN_POINT ( 'NONE',  ( 54.18750000000000711, 9.999999999999989342, 11.99999999999999467 ) ) ;
#22292=CARTESIAN_POINT ( 'NONE',  ( 55.46643183416158962, 7.028187705514638672, 13.68930817193508531 ) ) ;
#22294=CARTESIAN_POINT ( 'NONE',  ( 52.87500000000000711, 7.878679656440349177, 12.87867965644035984 ) ) ;
#22302=CARTESIAN_POINT ( 'NONE',  ( 58.65393183416157541, 6.971812294485357775, 16.17458954617365663 ) ) ;
#22319=CARTESIAN_POINT ( 'NONE',  ( 50.75231816583844591, 7.219692298483957771, 17.87654654797633924 ) ) ;
#22323=MANIFOLD_SOLID_BREP ( 'Cavity1', #17741 ) ;
#22339=CARTESIAN_POINT ( 'NONE',  ( 54.78356816583844591, 8.275094609561968184, 11.02818770551464667 ) ) ;
#22348=CARTESIAN_POINT ( 'NONE',  ( 53.59143183416158962, 11.72490539043799984, 11.02818770551463246 ) ) ;
#22357=CARTESIAN_POINT ( 'NONE',  ( 51.65625000000000711, 7.000000000000002665, 16.24264068711929099 ) ) ;
#22380=ADVANCED_FACE ( 'NONE', ( #15183 ), #22442, .T. ) ;
#22397=CARTESIAN_POINT ( 'NONE',  ( 56.15625000000002132, 6.000000000000004441, 16.65685424949239390 ) ) ;
#22407=CARTESIAN_POINT ( 'NONE',  ( 55.03125000000000000, 11.24264068711929276, 18.00000000000000355 ) ) ;
#22412=CARTESIAN_POINT ( 'NONE',  ( 55.74768183416157541, 7.830560233210222876, 17.07320092032950498 ) ) ;
#22421=CARTESIAN_POINT ( 'NONE',  ( 55.37268183416157541, 7.926799079670491466, 12.83056023321021755 ) ) ;
#22439=CARTESIAN_POINT ( 'NONE',  ( 55.06481816583844591, 6.999999999999998224, 15.06805114094563436 ) ) ;
#22442=PLANE ( 'NONE',  #11875 ) ;
#22468=CARTESIAN_POINT ( 'NONE',  ( 54.28125000000000000, 8.343145750507600766, 11.00000000000000533 ) ) ;
#22514=PRODUCT_DEFINITION_SHAPE ( 'NONE', 'NONE',  #6539 ) ;
#22518=CARTESIAN_POINT ( 'NONE',  ( 58.31250000000000000, 14.00000000000000000, 14.99999999999997691 ) ) ;
#22530=CARTESIAN_POINT ( 'NONE',  ( 56.43750000000000000, 10.00000000000000711, 17.99999999999999645 ) ) ;
#22540=CARTESIAN_POINT ( 'NONE',  ( 54.24768183416157541, 7.830560233210222876, 17.07320092032950498 ) ) ;
#22552=CARTESIAN_POINT ( 'NONE',  ( 51.18750000000000711, 9.999999999999989342, 11.99999999999999467 ) ) ;
#22560=DIRECTION ( 'NONE',  ( 0.000000000000000000, -0.7071067811865406894, 0.7071067811865545671 ) ) ;
#22576=CARTESIAN_POINT ( 'NONE',  ( 53.28356816583845301, 8.689308171935074654, 12.02818770551464489 ) ) ;
#22600=CARTESIAN_POINT ( 'NONE',  ( 57.75000000000000000, 7.171572875253819923, 17.82842712474619873 ) ) ;
#22649=CARTESIAN_POINT ( 'NONE',  ( 54.65625000000001421, 7.000000000000003553, 16.24264068711929099 ) ) ;
#22654=CARTESIAN_POINT ( 'NONE',  ( 58.65393183416157541, 6.971812294485357775, 16.17458954617365663 ) ) ;
#22664=CARTESIAN_POINT ( 'NONE',  ( 59.21643183416158962, 12.97181229448535689, 16.31069182806490758 ) ) ;
#22682=CARTESIAN_POINT ( 'NONE',  ( 56.65856816583844591, 7.028187705514647554, 16.31069182806492179 ) ) ;
#22699=CARTESIAN_POINT ( 'NONE',  ( 52.21875000000001421, 14.00000000000001066, 16.65685424949235482 ) ) ;
#22712=CARTESIAN_POINT ( 'NONE',  ( 54.93750000000000711, 10.00000000000001776, 18.99999999999999645 ) ) ;
#22771=CARTESIAN_POINT ( 'NONE',  ( 54.62268183416157541, 12.07320092032950676, 17.16943976678977180 ) ) ;
#22780=CARTESIAN_POINT ( 'NONE',  ( 57.71643183416158251, 12.97181229448535689, 16.31069182806490758 ) ) ;
#22792=CARTESIAN_POINT ( 'NONE',  ( 56.47106816583845301, 6.971812294485350670, 13.82541045382635403 ) ) ;
#22802=CARTESIAN_POINT ( 'NONE',  ( 52.81481816583844591, 12.99999999999999822, 14.93194885905435676 ) ) ;
#22827=CARTESIAN_POINT ( 'NONE',  ( 57.93750000000000000, 10.00000000000001776, 18.99999999999999645 ) ) ;
#22891=CARTESIAN_POINT ( 'NONE',  ( 58.74768183416157541, 7.123453452023678523, 17.78030770151605822 ) ) ;
#22902=CARTESIAN_POINT ( 'NONE',  ( 51.99768183416157541, 12.16943976678977535, 12.92679907967048614 ) ) ;
#22913=CARTESIAN_POINT ( 'NONE',  ( 56.00231816583843170, 12.07320092032949610, 12.83056023321021044 ) ) ;
#22921=VECTOR ( 'NONE', #16390, 1000.000000000000000 ) ;
#22926=CARTESIAN_POINT ( 'NONE',  ( 57.59606816583843880, 11.17458954617364242, 11.97181229448534800 ) ) ;
#22955=CARTESIAN_POINT ( 'NONE',  ( 56.06250000000000000, 5.999999999999996447, 15.00000000000001599 ) ) ;
#23007=CARTESIAN_POINT ( 'NONE',  ( 51.00000000000000711, 12.12132034355963484, 12.87867965644034740 ) ) ;
#23013=CARTESIAN_POINT ( 'NONE',  ( 57.62268183416157541, 12.78030770151606177, 17.87654654797631792 ) ) ;
#23014=CARTESIAN_POINT ( 'NONE',  ( 59.99999999999999289, 11.45040179400661096, 18.39307336842673735 ) ) ;
#23023=CARTESIAN_POINT ( 'NONE',  ( 55.18518183416157541, 10.06805114094562548, 11.99999999999999645 ) ) ;
#23032=CARTESIAN_POINT ( 'NONE',  ( 51.22106816583844591, 14.02818770551465377, 16.58880310854672757 ) ) ;
#23038=CARTESIAN_POINT ( 'NONE',  ( 57.46875000000000711, 6.999999999999992895, 13.75735931288071967 ) ) ;
#23041=CARTESIAN_POINT ( 'NONE',  ( 52.15856816583843880, 7.028187705514647554, 16.31069182806492179 ) ) ;
#23065=CARTESIAN_POINT ( 'NONE',  ( 52.40625000000000000, 13.99999999999999289, 13.34314575050759544 ) ) ;
#23083=CARTESIAN_POINT ( 'NONE',  ( 53.15625000000001421, 6.000000000000004441, 16.65685424949239390 ) ) ;
#23121=CARTESIAN_POINT ( 'NONE',  ( 60.00000000000004974, 13.87186598631677192, 14.01465949560290625 ) ) ;
#23132=CARTESIAN_POINT ( 'NONE',  ( 60.99768183416157541, 12.87654654797631792, 12.21969229848393113 ) ) ;
#23143=CARTESIAN_POINT ( 'NONE',  ( 51.12731816583844591, 12.87654654797634102, 17.78030770151602979 ) ) ;
#23152=CARTESIAN_POINT ( 'NONE',  ( 57.18750000000000000, 9.999999999999989342, 11.99999999999999467 ) ) ;
#23179=CARTESIAN_POINT ( 'NONE',  ( 55.72106816583844591, 14.02818770551465377, 16.58880310854672757 ) ) ;
#23196=CARTESIAN_POINT ( 'NONE',  ( 58.06481816583843170, 5.999999999999996447, 15.06805114094564502 ) ) ;
#23213=CARTESIAN_POINT ( 'NONE',  ( 59.43750000000000711, 10.00000000000000711, 17.99999999999999645 ) ) ;
#23237=CARTESIAN_POINT ( 'NONE',  ( 60.00000000000000711, 10.89310377415101350, 18.37602675929336016 ) ) ;
#23249=CARTESIAN_POINT ( 'NONE',  ( 55.09143183416158962, 11.31069182806491291, 12.02818770551463778 ) ) ;
#23262=CARTESIAN_POINT ( 'NONE',  ( 58.90856816583844591, 12.97181229448534978, 13.68930817193506755 ) ) ;
#23273=CARTESIAN_POINT ( 'NONE',  ( 57.00000000000000000, 12.12132034355963484, 12.87867965644034740 ) ) ;
#23275=CARTESIAN_POINT ( 'NONE',  ( 58.03125000000000711, 11.24264068711929276, 18.00000000000000355 ) ) ;
#23308=CARTESIAN_POINT ( 'NONE',  ( 51.18750000000000711, 9.999999999999978684, 10.99999999999999645 ) ) ;
#23323=CARTESIAN_POINT ( 'NONE',  ( 59.15625000000001421, 6.000000000000004441, 16.65685424949239390 ) ) ;
#23328=CARTESIAN_POINT ( 'NONE',  ( 52.40625000000000000, 13.99999999999999289, 13.34314575050759544 ) ) ;
#23347=CARTESIAN_POINT ( 'NONE',  ( 56.62500000000000000, 12.12132034355964727, 17.12132034355963484 ) ) ;
#23368=CARTESIAN_POINT ( 'NONE',  ( 60.00000000000000000, 13.47525482677739284, 13.02150377394223391 ) ) ;
#23378=CARTESIAN_POINT ( 'NONE',  ( 52.84143183416158251, 8.689308171935088865, 17.97181229448535689 ) ) ;
#23388=CARTESIAN_POINT ( 'NONE',  ( 50.47106816583844591, 6.971812294485350670, 13.82541045382635403 ) ) ;
#23394=CARTESIAN_POINT ( 'NONE',  ( 59.43750000000000711, 10.00000000000000711, 17.99999999999999645 ) ) ;
#23396=CARTESIAN_POINT ( 'NONE',  ( 51.31481816583844591, 12.99999999999999822, 14.93194885905435676 ) ) ;
#23426=CARTESIAN_POINT ( 'NONE',  ( 57.78356816583844591, 8.275094609561968184, 11.02818770551464667 ) ) ;
#23446=CARTESIAN_POINT ( 'NONE',  ( 58.53356816583845301, 11.72490539043803004, 18.97181229448534268 ) ) ;
#23453=CARTESIAN_POINT ( 'NONE',  ( 52.74768183416157541, 7.830560233210222876, 17.07320092032950498 ) ) ;
#23462=CARTESIAN_POINT ( 'NONE',  ( 57.37500000000000000, 7.878679656440349177, 12.87867965644035984 ) ) ;
#23480=CARTESIAN_POINT ( 'NONE',  ( 60.00000000000004974, 12.90160382567056274, 16.03866470743757588 ) ) ;
#23491=CARTESIAN_POINT ( 'NONE',  ( 53.96643183416157541, 6.028187705514633343, 13.27509460956200016 ) ) ;
#23500=CARTESIAN_POINT ( 'NONE',  ( 59.34375000000000711, 8.757359312880723223, 18.00000000000000355 ) ) ;
#23508=CARTESIAN_POINT ( 'NONE',  ( 54.37500000000000711, 7.878679656440349177, 12.87867965644035984 ) ) ;
#23510=CARTESIAN_POINT ( 'NONE',  ( 59.43750000000000711, 10.00000000000000711, 17.99999999999999645 ) ) ;
#23519=CARTESIAN_POINT ( 'NONE',  ( 53.15625000000001421, 7.000000000000003553, 16.24264068711929099 ) ) ;
#23544=CARTESIAN_POINT ( 'NONE',  ( 57.22106816583844591, 14.02818770551465377, 16.58880310854672757 ) ) ;
#23562=CARTESIAN_POINT ( 'NONE',  ( 57.56250000000000000, 5.999999999999996447, 15.00000000000001599 ) ) ;
#23566=CARTESIAN_POINT ( 'NONE',  ( 54.00000000000000711, 12.82842712474617741, 12.17157287525379239 ) ) ;
#23577=CARTESIAN_POINT ( 'NONE',  ( 51.99768183416157541, 12.16943976678977535, 12.92679907967048614 ) ) ;
#23584=CARTESIAN_POINT ( 'NONE',  ( 58.78125000000000711, 8.757359312880703683, 11.99999999999999822 ) ) ;
#23616=CARTESIAN_POINT ( 'NONE',  ( 52.74768183416157541, 7.123453452023678523, 17.78030770151605822 ) ) ;
#23619=ADVANCED_BREP_SHAPE_REPRESENTATION ( '', ( #22323, #7318 ), #9953 ) ;
#23625=CARTESIAN_POINT ( 'NONE',  ( 59.53125000000000000, 11.24264068711929276, 18.00000000000000355 ) ) ;
#23633=CARTESIAN_POINT ( 'NONE',  ( 51.28125000000000000, 8.757359312880703683, 11.99999999999999822 ) ) ;
#23637=CARTESIAN_POINT ( 'NONE',  ( 52.03124999999999289, 11.24264068711929276, 18.00000000000000355 ) ) ;
#23644=CARTESIAN_POINT ( 'NONE',  ( 55.96875000000000000, 6.999999999999992895, 13.75735931288071967 ) ) ;
#23657=CARTESIAN_POINT ( 'NONE',  ( 51.00000000000000711, 12.12132034355963484, 12.87867965644034740 ) ) ;
#23663=CARTESIAN_POINT ( 'NONE',  ( 52.81481816583844591, 14.00000000000000178, 14.93194885905434610 ) ) ;
#23680=CARTESIAN_POINT ( 'NONE',  ( 55.31250000000000711, 14.00000000000000000, 14.99999999999997691 ) ) ;
#23685=CARTESIAN_POINT ( 'NONE',  ( 53.56481816583844591, 5.999999999999996447, 15.06805114094564502 ) ) ;
#23694=CARTESIAN_POINT ( 'NONE',  ( 59.68518183416157541, 10.06805114094561659, 10.99999999999999645 ) ) ;
ENDSEC;
END-ISO-10303-21;
